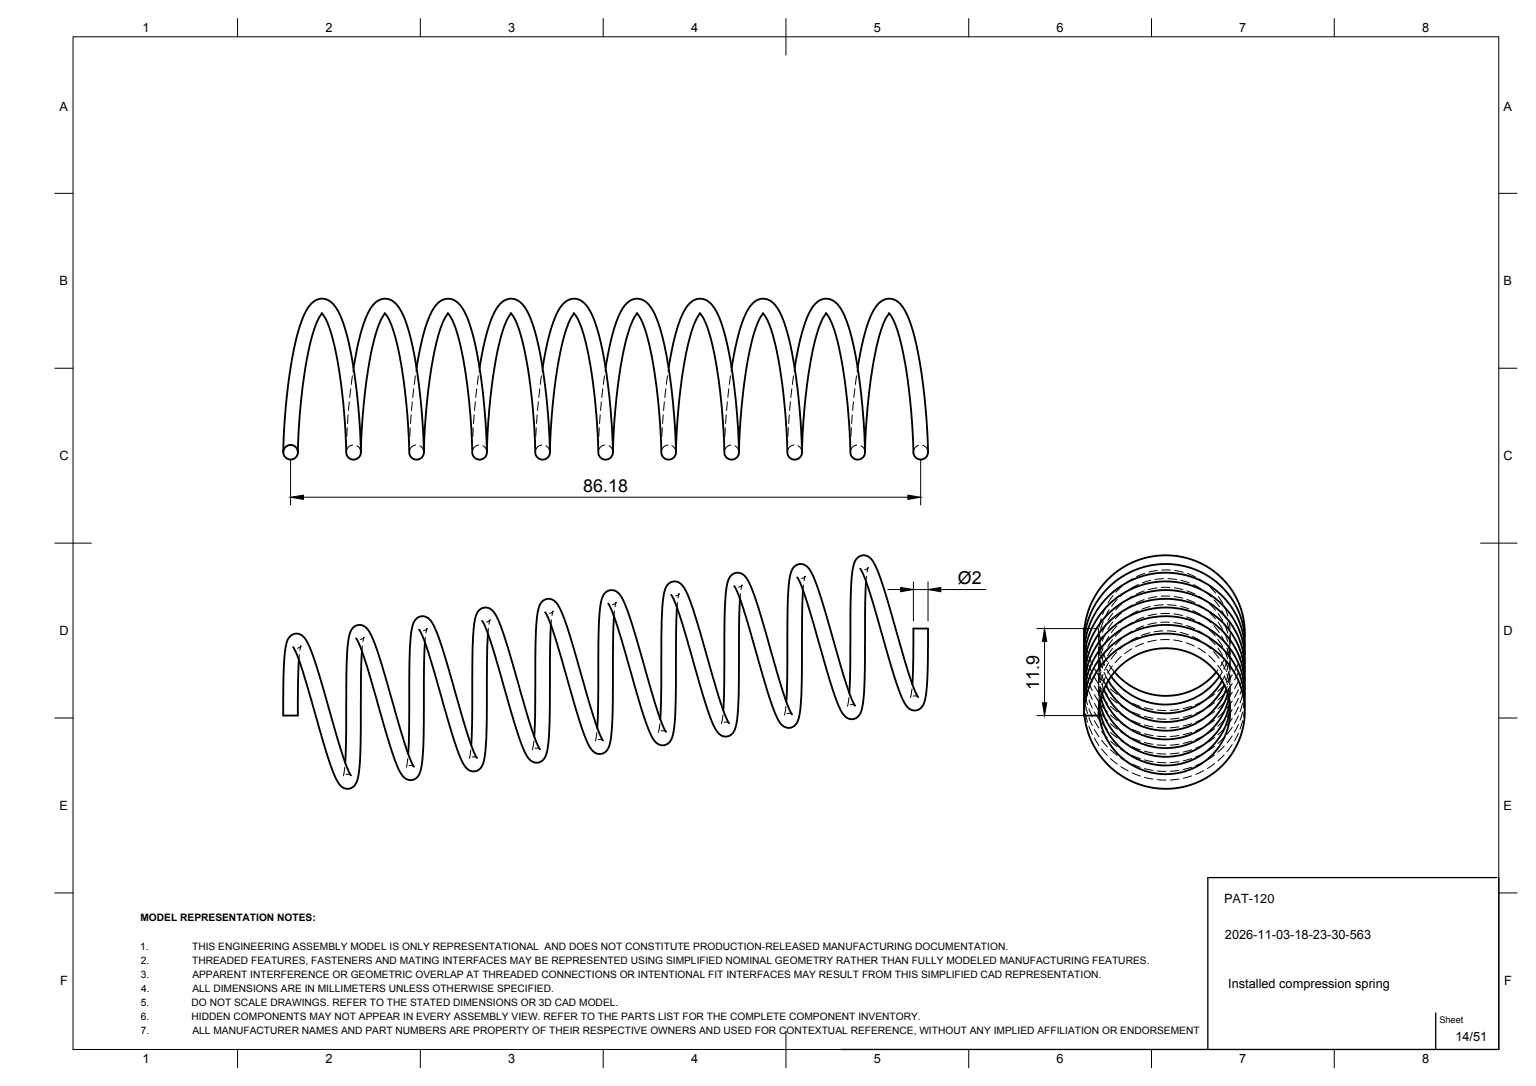
ISO-10303-21;
HEADER;
/* Generated by software containing ST-Developer
 * from STEP Tools, Inc. (www.steptools.com) 
 */

FILE_DESCRIPTION(
/* description */ ('Vibration shaker table dummy'),
/* implementation_level */ '2;1');

FILE_NAME(
/* name */ 'Installed compression spring.step',
/* time_stamp */ '2026-10-27T10:55:14-07:00',
/* author */ (''),
/* organization */ (''),
/* preprocessor_version */ 'ST-DEVELOPER v20.2',
/* originating_system */ 'Autodesk Translation Framework v15.17.0.0',
/* authorisation */ '');

FILE_SCHEMA (('AUTOMOTIVE_DESIGN { 1 0 10303 214 3 1 1 }'));
ENDSEC;

DATA;
#10=MECHANICAL_DESIGN_GEOMETRIC_PRESENTATION_REPRESENTATION('',(#695),#22394);
#586=B_SPLINE_CURVE_WITH_KNOTS('',3,(#15906,#15907,#15908,#15909,#15910,
#15911,#15912,#15913,#15914,#15915,#15916,#15917,#15918,#15919,#15920,#15921,
#15922,#15923,#15924,#15925,#15926,#15927,#15928,#15929,#15930,#15931,#15932,
#15933,#15934,#15935,#15936,#15937,#15938,#15939,#15940,#15941,#15942,#15943,
#15944,#15945,#15946,#15947,#15948,#15949,#15950,#15951,#15952,#15953,#15954,
#15955,#15956,#15957,#15958,#15959,#15960,#15961,#15962,#15963,#15964,#15965,
#15966,#15967,#15968,#15969,#15970,#15971,#15972,#15973,#15974,#15975,#15976,
#15977,#15978,#15979,#15980,#15981,#15982,#15983,#15984,#15985,#15986,#15987,
#15988,#15989,#15990,#15991,#15992,#15993,#15994,#15995,#15996,#15997,#15998,
#15999,#16000,#16001,#16002,#16003,#16004,#16005,#16006,#16007,#16008,#16009,
#16010,#16011,#16012,#16013,#16014,#16015,#16016,#16017,#16018,#16019,#16020,
#16021,#16022,#16023,#16024,#16025,#16026,#16027,#16028,#16029,#16030,#16031,
#16032,#16033,#16034,#16035,#16036,#16037,#16038,#16039),.UNSPECIFIED.,
 .F.,.F.,(4,1,1,1,1,1,1,1,1,1,1,1,1,1,1,1,1,1,1,1,1,1,1,1,1,1,1,1,1,1,1,
1,1,1,1,1,1,1,1,1,1,1,1,1,1,1,1,1,1,1,1,1,1,1,1,1,1,1,1,1,1,1,1,1,1,1,1,
1,1,1,1,1,1,1,1,1,1,1,1,1,1,1,1,1,1,1,1,1,1,1,1,1,1,1,1,1,1,1,1,1,1,1,1,
1,1,1,1,1,1,1,1,1,1,1,1,1,1,1,1,1,1,1,1,1,1,1,1,1,1,1,1,4),(0.,0.00892857142857143,
0.0178571428571429,0.0267857142857143,0.0357142857142857,0.0446428571428571,
0.0535714285714286,0.0625,0.0714285714285714,0.0803571428571428,0.0892857142857143,
0.0982142857142857,0.107142857142857,0.116071428571429,0.125,0.133928571428571,
0.142857142857143,0.150793650793651,0.154761904761905,0.156746031746032,
0.158730158730159,0.166666666666667,0.174603174603175,0.182539682539683,
0.19047619047619,0.196428571428571,0.202380952380952,0.208333333333333,
0.214285714285714,0.222222222222222,0.23015873015873,0.238095238095238,
0.241071428571429,0.244047619047619,0.25,0.255952380952381,0.261904761904762,
0.267857142857143,0.273809523809524,0.279761904761905,0.285714285714286,
0.297619047619048,0.30952380952381,0.321428571428571,0.327380952380952,
0.333333333333333,0.341269841269841,0.349206349206349,0.357142857142857,
0.365079365079365,0.373015873015873,0.380952380952381,0.386904761904762,
0.392857142857143,0.398809523809524,0.404761904761905,0.410714285714286,
0.416666666666667,0.422619047619048,0.428571428571429,0.4375,0.446428571428571,
0.455357142857143,0.459821428571429,0.464285714285714,0.470238095238095,
0.482142857142857,0.491071428571429,0.5,0.508928571428571,0.517857142857143,
0.526785714285714,0.535714285714286,0.544642857142857,0.553571428571429,
0.5625,0.571428571428571,0.580357142857143,0.589285714285714,0.598214285714286,
0.607142857142857,0.616071428571429,0.625,0.633928571428571,0.638392857142857,
0.642857142857143,0.650793650793651,0.658730158730159,0.666666666666667,
0.672619047619048,0.678571428571428,0.684523809523809,0.69047619047619,
0.696428571428571,0.702380952380952,0.708333333333333,0.714285714285714,
0.720238095238095,0.726190476190476,0.732142857142857,0.738095238095238,
0.744047619047619,0.75,0.755952380952381,0.761904761904762,0.76984126984127,
0.777777777777778,0.785714285714286,0.794642857142857,0.803571428571428,
0.8125,0.821428571428571,0.830357142857143,0.839285714285714,0.848214285714286,
0.857142857142857,0.866071428571429,0.875,0.883928571428571,0.892857142857143,
0.901785714285714,0.910714285714286,0.919642857142857,0.928571428571429,
0.9375,0.946428571428571,0.955357142857143,0.964285714285714,0.973214285714286,
0.982142857142857,0.991071428571429,1.),.UNSPECIFIED.);
#590=B_SPLINE_SURFACE_WITH_KNOTS('',3,3,((#14563,#14564,#14565,#14566,#14567,
#14568,#14569,#14570,#14571,#14572,#14573,#14574,#14575,#14576,#14577,#14578,
#14579,#14580,#14581,#14582,#14583,#14584,#14585,#14586,#14587,#14588,#14589,
#14590,#14591,#14592,#14593,#14594,#14595,#14596,#14597,#14598,#14599,#14600,
#14601,#14602,#14603,#14604,#14605,#14606,#14607,#14608,#14609,#14610,#14611,
#14612,#14613,#14614,#14615,#14616,#14617,#14618,#14619,#14620,#14621,#14622,
#14623,#14624,#14625,#14626,#14627,#14628,#14629,#14630,#14631,#14632,#14633,
#14634,#14635,#14636,#14637,#14638,#14639,#14640,#14641,#14642,#14643,#14644,
#14645,#14646,#14647,#14648,#14649,#14650,#14651,#14652,#14653,#14654,#14655,
#14656,#14657,#14658,#14659,#14660,#14661,#14662,#14663,#14664,#14665,#14666,
#14667,#14668,#14669,#14670,#14671,#14672,#14673,#14674,#14675,#14676,#14677,
#14678,#14679,#14680,#14681,#14682,#14683,#14684,#14685,#14686,#14687,#14688,
#14689,#14690,#14691,#14692,#14693,#14694,#14695,#14696),(#14697,#14698,
#14699,#14700,#14701,#14702,#14703,#14704,#14705,#14706,#14707,#14708,#14709,
#14710,#14711,#14712,#14713,#14714,#14715,#14716,#14717,#14718,#14719,#14720,
#14721,#14722,#14723,#14724,#14725,#14726,#14727,#14728,#14729,#14730,#14731,
#14732,#14733,#14734,#14735,#14736,#14737,#14738,#14739,#14740,#14741,#14742,
#14743,#14744,#14745,#14746,#14747,#14748,#14749,#14750,#14751,#14752,#14753,
#14754,#14755,#14756,#14757,#14758,#14759,#14760,#14761,#14762,#14763,#14764,
#14765,#14766,#14767,#14768,#14769,#14770,#14771,#14772,#14773,#14774,#14775,
#14776,#14777,#14778,#14779,#14780,#14781,#14782,#14783,#14784,#14785,#14786,
#14787,#14788,#14789,#14790,#14791,#14792,#14793,#14794,#14795,#14796,#14797,
#14798,#14799,#14800,#14801,#14802,#14803,#14804,#14805,#14806,#14807,#14808,
#14809,#14810,#14811,#14812,#14813,#14814,#14815,#14816,#14817,#14818,#14819,
#14820,#14821,#14822,#14823,#14824,#14825,#14826,#14827,#14828,#14829,#14830),
(#14831,#14832,#14833,#14834,#14835,#14836,#14837,#14838,#14839,#14840,
#14841,#14842,#14843,#14844,#14845,#14846,#14847,#14848,#14849,#14850,#14851,
#14852,#14853,#14854,#14855,#14856,#14857,#14858,#14859,#14860,#14861,#14862,
#14863,#14864,#14865,#14866,#14867,#14868,#14869,#14870,#14871,#14872,#14873,
#14874,#14875,#14876,#14877,#14878,#14879,#14880,#14881,#14882,#14883,#14884,
#14885,#14886,#14887,#14888,#14889,#14890,#14891,#14892,#14893,#14894,#14895,
#14896,#14897,#14898,#14899,#14900,#14901,#14902,#14903,#14904,#14905,#14906,
#14907,#14908,#14909,#14910,#14911,#14912,#14913,#14914,#14915,#14916,#14917,
#14918,#14919,#14920,#14921,#14922,#14923,#14924,#14925,#14926,#14927,#14928,
#14929,#14930,#14931,#14932,#14933,#14934,#14935,#14936,#14937,#14938,#14939,
#14940,#14941,#14942,#14943,#14944,#14945,#14946,#14947,#14948,#14949,#14950,
#14951,#14952,#14953,#14954,#14955,#14956,#14957,#14958,#14959,#14960,#14961,
#14962,#14963,#14964),(#14965,#14966,#14967,#14968,#14969,#14970,#14971,
#14972,#14973,#14974,#14975,#14976,#14977,#14978,#14979,#14980,#14981,#14982,
#14983,#14984,#14985,#14986,#14987,#14988,#14989,#14990,#14991,#14992,#14993,
#14994,#14995,#14996,#14997,#14998,#14999,#15000,#15001,#15002,#15003,#15004,
#15005,#15006,#15007,#15008,#15009,#15010,#15011,#15012,#15013,#15014,#15015,
#15016,#15017,#15018,#15019,#15020,#15021,#15022,#15023,#15024,#15025,#15026,
#15027,#15028,#15029,#15030,#15031,#15032,#15033,#15034,#15035,#15036,#15037,
#15038,#15039,#15040,#15041,#15042,#15043,#15044,#15045,#15046,#15047,#15048,
#15049,#15050,#15051,#15052,#15053,#15054,#15055,#15056,#15057,#15058,#15059,
#15060,#15061,#15062,#15063,#15064,#15065,#15066,#15067,#15068,#15069,#15070,
#15071,#15072,#15073,#15074,#15075,#15076,#15077,#15078,#15079,#15080,#15081,
#15082,#15083,#15084,#15085,#15086,#15087,#15088,#15089,#15090,#15091,#15092,
#15093,#15094,#15095,#15096,#15097,#15098),(#15099,#15100,#15101,#15102,
#15103,#15104,#15105,#15106,#15107,#15108,#15109,#15110,#15111,#15112,#15113,
#15114,#15115,#15116,#15117,#15118,#15119,#15120,#15121,#15122,#15123,#15124,
#15125,#15126,#15127,#15128,#15129,#15130,#15131,#15132,#15133,#15134,#15135,
#15136,#15137,#15138,#15139,#15140,#15141,#15142,#15143,#15144,#15145,#15146,
#15147,#15148,#15149,#15150,#15151,#15152,#15153,#15154,#15155,#15156,#15157,
#15158,#15159,#15160,#15161,#15162,#15163,#15164,#15165,#15166,#15167,#15168,
#15169,#15170,#15171,#15172,#15173,#15174,#15175,#15176,#15177,#15178,#15179,
#15180,#15181,#15182,#15183,#15184,#15185,#15186,#15187,#15188,#15189,#15190,
#15191,#15192,#15193,#15194,#15195,#15196,#15197,#15198,#15199,#15200,#15201,
#15202,#15203,#15204,#15205,#15206,#15207,#15208,#15209,#15210,#15211,#15212,
#15213,#15214,#15215,#15216,#15217,#15218,#15219,#15220,#15221,#15222,#15223,
#15224,#15225,#15226,#15227,#15228,#15229,#15230,#15231,#15232),(#15233,
#15234,#15235,#15236,#15237,#15238,#15239,#15240,#15241,#15242,#15243,#15244,
#15245,#15246,#15247,#15248,#15249,#15250,#15251,#15252,#15253,#15254,#15255,
#15256,#15257,#15258,#15259,#15260,#15261,#15262,#15263,#15264,#15265,#15266,
#15267,#15268,#15269,#15270,#15271,#15272,#15273,#15274,#15275,#15276,#15277,
#15278,#15279,#15280,#15281,#15282,#15283,#15284,#15285,#15286,#15287,#15288,
#15289,#15290,#15291,#15292,#15293,#15294,#15295,#15296,#15297,#15298,#15299,
#15300,#15301,#15302,#15303,#15304,#15305,#15306,#15307,#15308,#15309,#15310,
#15311,#15312,#15313,#15314,#15315,#15316,#15317,#15318,#15319,#15320,#15321,
#15322,#15323,#15324,#15325,#15326,#15327,#15328,#15329,#15330,#15331,#15332,
#15333,#15334,#15335,#15336,#15337,#15338,#15339,#15340,#15341,#15342,#15343,
#15344,#15345,#15346,#15347,#15348,#15349,#15350,#15351,#15352,#15353,#15354,
#15355,#15356,#15357,#15358,#15359,#15360,#15361,#15362,#15363,#15364,#15365,
#15366),(#15367,#15368,#15369,#15370,#15371,#15372,#15373,#15374,#15375,
#15376,#15377,#15378,#15379,#15380,#15381,#15382,#15383,#15384,#15385,#15386,
#15387,#15388,#15389,#15390,#15391,#15392,#15393,#15394,#15395,#15396,#15397,
#15398,#15399,#15400,#15401,#15402,#15403,#15404,#15405,#15406,#15407,#15408,
#15409,#15410,#15411,#15412,#15413,#15414,#15415,#15416,#15417,#15418,#15419,
#15420,#15421,#15422,#15423,#15424,#15425,#15426,#15427,#15428,#15429,#15430,
#15431,#15432,#15433,#15434,#15435,#15436,#15437,#15438,#15439,#15440,#15441,
#15442,#15443,#15444,#15445,#15446,#15447,#15448,#15449,#15450,#15451,#15452,
#15453,#15454,#15455,#15456,#15457,#15458,#15459,#15460,#15461,#15462,#15463,
#15464,#15465,#15466,#15467,#15468,#15469,#15470,#15471,#15472,#15473,#15474,
#15475,#15476,#15477,#15478,#15479,#15480,#15481,#15482,#15483,#15484,#15485,
#15486,#15487,#15488,#15489,#15490,#15491,#15492,#15493,#15494,#15495,#15496,
#15497,#15498,#15499,#15500),(#15501,#15502,#15503,#15504,#15505,#15506,
#15507,#15508,#15509,#15510,#15511,#15512,#15513,#15514,#15515,#15516,#15517,
#15518,#15519,#15520,#15521,#15522,#15523,#15524,#15525,#15526,#15527,#15528,
#15529,#15530,#15531,#15532,#15533,#15534,#15535,#15536,#15537,#15538,#15539,
#15540,#15541,#15542,#15543,#15544,#15545,#15546,#15547,#15548,#15549,#15550,
#15551,#15552,#15553,#15554,#15555,#15556,#15557,#15558,#15559,#15560,#15561,
#15562,#15563,#15564,#15565,#15566,#15567,#15568,#15569,#15570,#15571,#15572,
#15573,#15574,#15575,#15576,#15577,#15578,#15579,#15580,#15581,#15582,#15583,
#15584,#15585,#15586,#15587,#15588,#15589,#15590,#15591,#15592,#15593,#15594,
#15595,#15596,#15597,#15598,#15599,#15600,#15601,#15602,#15603,#15604,#15605,
#15606,#15607,#15608,#15609,#15610,#15611,#15612,#15613,#15614,#15615,#15616,
#15617,#15618,#15619,#15620,#15621,#15622,#15623,#15624,#15625,#15626,#15627,
#15628,#15629,#15630,#15631,#15632,#15633,#15634),(#15635,#15636,#15637,
#15638,#15639,#15640,#15641,#15642,#15643,#15644,#15645,#15646,#15647,#15648,
#15649,#15650,#15651,#15652,#15653,#15654,#15655,#15656,#15657,#15658,#15659,
#15660,#15661,#15662,#15663,#15664,#15665,#15666,#15667,#15668,#15669,#15670,
#15671,#15672,#15673,#15674,#15675,#15676,#15677,#15678,#15679,#15680,#15681,
#15682,#15683,#15684,#15685,#15686,#15687,#15688,#15689,#15690,#15691,#15692,
#15693,#15694,#15695,#15696,#15697,#15698,#15699,#15700,#15701,#15702,#15703,
#15704,#15705,#15706,#15707,#15708,#15709,#15710,#15711,#15712,#15713,#15714,
#15715,#15716,#15717,#15718,#15719,#15720,#15721,#15722,#15723,#15724,#15725,
#15726,#15727,#15728,#15729,#15730,#15731,#15732,#15733,#15734,#15735,#15736,
#15737,#15738,#15739,#15740,#15741,#15742,#15743,#15744,#15745,#15746,#15747,
#15748,#15749,#15750,#15751,#15752,#15753,#15754,#15755,#15756,#15757,#15758,
#15759,#15760,#15761,#15762,#15763,#15764,#15765,#15766,#15767,#15768),
(#15769,#15770,#15771,#15772,#15773,#15774,#15775,#15776,#15777,#15778,
#15779,#15780,#15781,#15782,#15783,#15784,#15785,#15786,#15787,#15788,#15789,
#15790,#15791,#15792,#15793,#15794,#15795,#15796,#15797,#15798,#15799,#15800,
#15801,#15802,#15803,#15804,#15805,#15806,#15807,#15808,#15809,#15810,#15811,
#15812,#15813,#15814,#15815,#15816,#15817,#15818,#15819,#15820,#15821,#15822,
#15823,#15824,#15825,#15826,#15827,#15828,#15829,#15830,#15831,#15832,#15833,
#15834,#15835,#15836,#15837,#15838,#15839,#15840,#15841,#15842,#15843,#15844,
#15845,#15846,#15847,#15848,#15849,#15850,#15851,#15852,#15853,#15854,#15855,
#15856,#15857,#15858,#15859,#15860,#15861,#15862,#15863,#15864,#15865,#15866,
#15867,#15868,#15869,#15870,#15871,#15872,#15873,#15874,#15875,#15876,#15877,
#15878,#15879,#15880,#15881,#15882,#15883,#15884,#15885,#15886,#15887,#15888,
#15889,#15890,#15891,#15892,#15893,#15894,#15895,#15896,#15897,#15898,#15899,
#15900,#15901,#15902)),.UNSPECIFIED.,.T.,.F.,.F.,(4,1,1,1,1,1,1,4),(4,1,
1,1,1,1,1,1,1,1,1,1,1,1,1,1,1,1,1,1,1,1,1,1,1,1,1,1,1,1,1,1,1,1,1,1,1,1,
1,1,1,1,1,1,1,1,1,1,1,1,1,1,1,1,1,1,1,1,1,1,1,1,1,1,1,1,1,1,1,1,1,1,1,1,
1,1,1,1,1,1,1,1,1,1,1,1,1,1,1,1,1,1,1,1,1,1,1,1,1,1,1,1,1,1,1,1,1,1,1,1,
1,1,1,1,1,1,1,1,1,1,1,1,1,1,1,1,1,1,1,1,1,4),(-3.14159265358979,-2.24399475256414,
-1.34639685153848,-0.448798950512828,0.448798950512828,1.34639685153848,
2.24399475256414,3.14159265358979),(0.,0.00892857142857143,0.0178571428571429,
0.0267857142857143,0.0357142857142857,0.0446428571428571,0.0535714285714286,
0.0625,0.0714285714285714,0.0803571428571428,0.0892857142857143,0.0982142857142857,
0.107142857142857,0.116071428571429,0.125,0.133928571428571,0.142857142857143,
0.150793650793651,0.154761904761905,0.156746031746032,0.158730158730159,
0.166666666666667,0.174603174603175,0.182539682539683,0.19047619047619,
0.196428571428571,0.202380952380952,0.208333333333333,0.214285714285714,
0.222222222222222,0.23015873015873,0.238095238095238,0.241071428571429,
0.244047619047619,0.25,0.255952380952381,0.261904761904762,0.267857142857143,
0.273809523809524,0.279761904761905,0.285714285714286,0.297619047619048,
0.30952380952381,0.321428571428571,0.327380952380952,0.333333333333333,
0.341269841269841,0.349206349206349,0.357142857142857,0.365079365079365,
0.373015873015873,0.380952380952381,0.386904761904762,0.392857142857143,
0.398809523809524,0.404761904761905,0.410714285714286,0.416666666666667,
0.422619047619048,0.428571428571429,0.4375,0.446428571428571,0.455357142857143,
0.459821428571429,0.464285714285714,0.470238095238095,0.482142857142857,
0.491071428571429,0.5,0.508928571428571,0.517857142857143,0.526785714285714,
0.535714285714286,0.544642857142857,0.553571428571429,0.5625,0.571428571428571,
0.580357142857143,0.589285714285714,0.598214285714286,0.607142857142857,
0.616071428571429,0.625,0.633928571428571,0.638392857142857,0.642857142857143,
0.650793650793651,0.658730158730159,0.666666666666667,0.672619047619048,
0.678571428571428,0.684523809523809,0.69047619047619,0.696428571428571,
0.702380952380952,0.708333333333333,0.714285714285714,0.720238095238095,
0.726190476190476,0.732142857142857,0.738095238095238,0.744047619047619,
0.75,0.755952380952381,0.761904761904762,0.76984126984127,0.777777777777778,
0.785714285714286,0.794642857142857,0.803571428571428,0.8125,0.821428571428571,
0.830357142857143,0.839285714285714,0.848214285714286,0.857142857142857,
0.866071428571429,0.875,0.883928571428571,0.892857142857143,0.901785714285714,
0.910714285714286,0.919642857142857,0.928571428571429,0.9375,0.946428571428571,
0.955357142857143,0.964285714285714,0.973214285714286,0.982142857142857,
0.991071428571429,1.),.UNSPECIFIED.);
#603=SHAPE_REPRESENTATION_RELATIONSHIP('SRR','None',#22649,#649);
#649=ADVANCED_BREP_SHAPE_REPRESENTATION('',(#741),#22355);
#695=STYLED_ITEM('',(#22961),#741);
#741=MANIFOLD_SOLID_BREP('Body1',#9213);
#1124=PLANE('',#10016);
#1125=PLANE('',#10017);
#1463=FACE_OUTER_BOUND('',#2063,.T.);
#1464=FACE_OUTER_BOUND('',#2064,.T.);
#1465=FACE_OUTER_BOUND('',#2065,.T.);
#2063=EDGE_LOOP('',(#6822,#6823,#6824,#6825));
#2064=EDGE_LOOP('',(#6826));
#2065=EDGE_LOOP('',(#6827));
#3980=CIRCLE('',#10014,0.1);
#3981=CIRCLE('',#10015,0.1);
#4559=VERTEX_POINT('',#15903);
#4560=VERTEX_POINT('',#15905);
#5404=EDGE_CURVE('',#4559,#4559,#3980,.T.);
#5405=EDGE_CURVE('',#4559,#4560,#586,.T.);
#5406=EDGE_CURVE('',#4560,#4560,#3981,.T.);
#6822=ORIENTED_EDGE('',*,*,#5404,.T.);
#6823=ORIENTED_EDGE('',*,*,#5405,.T.);
#6824=ORIENTED_EDGE('',*,*,#5406,.F.);
#6825=ORIENTED_EDGE('',*,*,#5405,.F.);
#6826=ORIENTED_EDGE('',*,*,#5406,.T.);
#6827=ORIENTED_EDGE('',*,*,#5404,.F.);
#8828=ADVANCED_FACE('',(#1463),#590,.T.);
#8829=ADVANCED_FACE('',(#1464),#1124,.T.);
#8830=ADVANCED_FACE('',(#1465),#1125,.F.);
#9213=CLOSED_SHELL('',(#8828,#8829,#8830));
#10013=AXIS2_PLACEMENT_3D('',#14562,#11624,#11625);
#10014=AXIS2_PLACEMENT_3D('',#15904,#11626,#11627);
#10015=AXIS2_PLACEMENT_3D('',#16040,#11628,#11629);
#10016=AXIS2_PLACEMENT_3D('',#16041,#11630,#11631);
#10017=AXIS2_PLACEMENT_3D('',#16042,#11632,#11633);
#11624=DIRECTION('axis',(0.,0.,1.));
#11625=DIRECTION('refdir',(1.,0.,0.));
#11626=DIRECTION('center_axis',(-0.000133356290274077,0.990604928518996,
0.136754735969086));
#11627=DIRECTION('ref_axis',(1.84100680060121E-5,-0.136754734729895,0.990604937495279));
#11628=DIRECTION('center_axis',(0.000133356194773129,0.99060492849245,0.136754736161472));
#11629=DIRECTION('ref_axis',(-0.722226697925938,0.0946826990450871,-0.685145081938514));
#11630=DIRECTION('center_axis',(0.000133356194773129,0.99060492849245,0.136754736161472));
#11631=DIRECTION('ref_axis',(-0.722226697925938,0.0946826990450871,-0.685145081938514));
#11632=DIRECTION('center_axis',(-0.000133356290274077,0.990604928518996,
0.136754735969086));
#11633=DIRECTION('ref_axis',(1.84100680060121E-5,-0.136754734729895,0.990604937495279));
#14562=CARTESIAN_POINT('',(0.,0.,0.));
#14563=CARTESIAN_POINT('Ctrl Pts',(-5.0000018410068,-3.98632452652701,2.60093950625047));
#14564=CARTESIAN_POINT('Ctrl Pts',(-5.00002711936198,-3.79855038268961,
2.62686205390092));
#14565=CARTESIAN_POINT('Ctrl Pts',(-5.10766548646186,-3.42414266353048,
2.67881373981085));
#14566=CARTESIAN_POINT('Ctrl Pts',(-5.54728618664091,-3.02997941177219,
2.75738438838345));
#14567=CARTESIAN_POINT('Ctrl Pts',(-6.13328094577175,-2.93005881251319,
2.83651316903494));
#14568=CARTESIAN_POINT('Ctrl Pts',(-6.68670283260197,-3.15858336118752,
2.91622304878198));
#14569=CARTESIAN_POINT('Ctrl Pts',(-7.03616187921695,-3.65012597802659,
2.99648821676135));
#14570=CARTESIAN_POINT('Ctrl Pts',(-7.07062949516082,-4.25616589762635,
3.07729930317819));
#14571=CARTESIAN_POINT('Ctrl Pts',(-6.77580863517498,-4.79139923899731,
3.15863489698049));
#14572=CARTESIAN_POINT('Ctrl Pts',(-6.23777999713871,-5.08919902934938,
3.24047455745509));
#14573=CARTESIAN_POINT('Ctrl Pts',(-5.62032344264714,-5.05504677509261,
3.32279321070673));
#14574=CARTESIAN_POINT('Ctrl Pts',(-5.11287137916696,-4.69557478020053,
3.40556356877954));
#14575=CARTESIAN_POINT('Ctrl Pts',(-4.87329914702911,-4.11831903637453,
3.48875540125931));
#14576=CARTESIAN_POINT('Ctrl Pts',(-4.97807346419814,-3.49920456570944,
3.57233609900605));
#14577=CARTESIAN_POINT('Ctrl Pts',(-5.39799493781825,-3.02877333945258,
3.65627071903615));
#14578=CARTESIAN_POINT('Ctrl Pts',(-6.00610273172108,-2.85326324045065,
3.74052224127624));
#14579=CARTESIAN_POINT('Ctrl Pts',(-6.61643757836359,-3.02876545098225,
3.82505176791358));
#14580=CARTESIAN_POINT('Ctrl Pts',(-7.02513160270699,-3.48597574268572,
3.90667922493066));
#14581=CARTESIAN_POINT('Ctrl Pts',(-7.12235641775929,-3.9685483460108,3.97275270898905));
#14582=CARTESIAN_POINT('Ctrl Pts',(-7.06636481269846,-4.28466100128236,
4.01685604551847));
#14583=CARTESIAN_POINT('Ctrl Pts',(-7.00182040328561,-4.45530975229043,
4.04207155819959));
#14584=CARTESIAN_POINT('Ctrl Pts',(-6.87402691871924,-4.69744869614318,
4.07990746733096));
#14585=CARTESIAN_POINT('Ctrl Pts',(-6.57124878899927,-4.99309357202046,
4.1367051149187));
#14586=CARTESIAN_POINT('Ctrl Pts',(-6.02768033690931,-5.14605913758532,
4.2124974864954));
#14587=CARTESIAN_POINT('Ctrl Pts',(-5.47679456345111,-5.0204436702095,4.28832048286543));
#14588=CARTESIAN_POINT('Ctrl Pts',(-5.08889541312948,-4.67743201497751,
4.35782392862843));
#14589=CARTESIAN_POINT('Ctrl Pts',(-4.90355272665998,-4.25185719379132,
4.42098501738742));
#14590=CARTESIAN_POINT('Ctrl Pts',(-4.88772422317122,-3.83457870292561,
4.47779828347438));
#14591=CARTESIAN_POINT('Ctrl Pts',(-5.02577825319216,-3.44096047951616,
4.5345666000236));
#14592=CARTESIAN_POINT('Ctrl Pts',(-5.32758243531257,-3.08955719770179,
4.59757801626674));
#14593=CARTESIAN_POINT('Ctrl Pts',(-5.79757132369034,-2.87764760865861,
4.66678930745632));
#14594=CARTESIAN_POINT('Ctrl Pts',(-6.35748141231083,-2.91980778121556,
4.74213608943437));
#14595=CARTESIAN_POINT('Ctrl Pts',(-6.72958410590507,-3.16055362161142,
4.80163845366161));
#14596=CARTESIAN_POINT('Ctrl Pts',(-6.922583408066,-3.41255717151317,4.8453962925926));
#14597=CARTESIAN_POINT('Ctrl Pts',(-7.04520229026909,-3.65506744231538,
4.88286085267916));
#14598=CARTESIAN_POINT('Ctrl Pts',(-7.10903827020174,-3.9926759490213,4.92960885619655));
#14599=CARTESIAN_POINT('Ctrl Pts',(-7.032354492376,-4.39667067923105,4.98556279568034));
#14600=CARTESIAN_POINT('Ctrl Pts',(-6.81415974257675,-4.74396102273289,
5.04136211338037));
#14601=CARTESIAN_POINT('Ctrl Pts',(-6.48510242262688,-4.98648342248571,
5.09699623581333));
#14602=CARTESIAN_POINT('Ctrl Pts',(-6.09122164110091,-5.09213718968761,
5.15245506498449));
#14603=CARTESIAN_POINT('Ctrl Pts',(-5.6879156360413,-5.04618557814476,5.20772889788153));
#14604=CARTESIAN_POINT('Ctrl Pts',(-5.20960410281967,-4.79482820495352,
5.28116853491036));
#14605=CARTESIAN_POINT('Ctrl Pts',(-4.85635661256684,-4.18339627204868,
5.37246079310469));
#14606=CARTESIAN_POINT('Ctrl Pts',(-5.04534497366866,-3.36152922837358,
5.4811368047244));
#14607=CARTESIAN_POINT('Ctrl Pts',(-5.62045222073828,-2.97210695679973,
5.57092649482181));
#14608=CARTESIAN_POINT('Ctrl Pts',(-6.14491401311764,-2.95446524901901,
5.64227218329944));
#14609=CARTESIAN_POINT('Ctrl Pts',(-6.55538629310792,-3.09741218079302,
5.70145206897501));
#14610=CARTESIAN_POINT('Ctrl Pts',(-6.90061904209687,-3.43455608810828,
5.76619150175189));
#14611=CARTESIAN_POINT('Ctrl Pts',(-7.05403180026006,-3.93434682913999,
5.83636208061574));
#14612=CARTESIAN_POINT('Ctrl Pts',(-6.95084370870626,-4.44331194962687,
5.90607316768221));
#14613=CARTESIAN_POINT('Ctrl Pts',(-6.61884201115902,-4.83828819326241,
5.97532164622816));
#14614=CARTESIAN_POINT('Ctrl Pts',(-6.14163977231472,-5.02507153362565,
6.04410658214742));
#14615=CARTESIAN_POINT('Ctrl Pts',(-5.67874308979945,-4.96670943531882,
6.10673565115305));
#14616=CARTESIAN_POINT('Ctrl Pts',(-5.32673727495899,-4.74487796933182,
6.16333654805419));
#14617=CARTESIAN_POINT('Ctrl Pts',(-5.10557737295403,-4.44521639081723,
6.21402149420468));
#14618=CARTESIAN_POINT('Ctrl Pts',(-5.00986236436416,-4.08706033297606,
6.26445344628883));
#14619=CARTESIAN_POINT('Ctrl Pts',(-5.05132140869747,-3.72058500062059,
6.31463598386295));
#14620=CARTESIAN_POINT('Ctrl Pts',(-5.22295427342147,-3.39619318419661,
6.36457331207659));
#14621=CARTESIAN_POINT('Ctrl Pts',(-5.49996349858563,-3.15797332202467,
6.41427030413784));
#14622=CARTESIAN_POINT('Ctrl Pts',(-5.843023257891,-3.03825996963253,6.46373244033231));
#14623=CARTESIAN_POINT('Ctrl Pts',(-6.2651798733637,-3.05368284090179,6.52117143934356));
#14624=CARTESIAN_POINT('Ctrl Pts',(-6.69395218073661,-3.29085487418832,
6.58644589644131));
#14625=CARTESIAN_POINT('Ctrl Pts',(-6.9588514090406,-3.77142724594311,6.65940509135759));
#14626=CARTESIAN_POINT('Ctrl Pts',(-6.93289301903251,-4.22410112506723,
6.71983222544231));
#14627=CARTESIAN_POINT('Ctrl Pts',(-6.77106481048377,-4.53615877260298,
6.76796591761938));
#14628=CARTESIAN_POINT('Ctrl Pts',(-6.57088599598262,-4.74749645053629,
6.8079662999785));
#14629=CARTESIAN_POINT('Ctrl Pts',(-6.18196007039062,-4.95496402481898,
6.86778079666891));
#14630=CARTESIAN_POINT('Ctrl Pts',(-5.63200940413013,-4.91297894303413,
6.93919834468442));
#14631=CARTESIAN_POINT('Ctrl Pts',(-5.18963313111942,-4.51545599119052,
7.01814869825501));
#14632=CARTESIAN_POINT('Ctrl Pts',(-5.04266994609727,-4.00519996765647,
7.08893288548598));
#14633=CARTESIAN_POINT('Ctrl Pts',(-5.18994160065279,-3.49569082009585,
7.15948665627275));
#14634=CARTESIAN_POINT('Ctrl Pts',(-5.58406477811046,-3.14370617953113,
7.22985222522876));
#14635=CARTESIAN_POINT('Ctrl Pts',(-6.10419876841606,-3.05543002721108,
7.30007283323036));
#14636=CARTESIAN_POINT('Ctrl Pts',(-6.59085610258569,-3.25712241290123,
7.37019262147636));
#14637=CARTESIAN_POINT('Ctrl Pts',(-6.8952969281062,-3.68642062054244,7.44025632508636));
#14638=CARTESIAN_POINT('Ctrl Pts',(-6.92507910037993,-4.2118623997588,7.51030900497373));
#14639=CARTESIAN_POINT('Ctrl Pts',(-6.67029196164112,-4.6727438878236,7.58039577683535));
#14640=CARTESIAN_POINT('Ctrl Pts',(-6.20902606294958,-4.92782413963266,
7.65056157433059));
#14641=CARTESIAN_POINT('Ctrl Pts',(-5.68175068955988,-4.89838259463549,
7.72085085746158));
#14642=CARTESIAN_POINT('Ctrl Pts',(-5.24995696526907,-4.59224234497362,
7.79130734612191));
#14643=CARTESIAN_POINT('Ctrl Pts',(-5.04653976812282,-4.10189023096155,
7.86197377554524));
#14644=CARTESIAN_POINT('Ctrl Pts',(-5.13553771446182,-3.57654536818086,
7.93289164421975));
#14645=CARTESIAN_POINT('Ctrl Pts',(-5.49167958880606,-3.17757206270347,
8.00410097016463));
#14646=CARTESIAN_POINT('Ctrl Pts',(-6.00820878856796,-3.02820291673281,
8.07564000225066));
#14647=CARTESIAN_POINT('Ctrl Pts',(-6.44062187419601,-3.15261370888403,
8.13556092469148));
#14648=CARTESIAN_POINT('Ctrl Pts',(-6.70861130655355,-3.37965195671477,
8.18369776363854));
#14649=CARTESIAN_POINT('Ctrl Pts',(-6.8937105085998,-3.65581236490976,8.22929135600403));
#14650=CARTESIAN_POINT('Ctrl Pts',(-6.97571459288556,-4.05892831151958,
8.28449961702882));
#14651=CARTESIAN_POINT('Ctrl Pts',(-6.83301647708075,-4.52172879570838,
8.34949564023339));
#14652=CARTESIAN_POINT('Ctrl Pts',(-6.51381452164907,-4.83374162454526,
8.40942447333573));
#14653=CARTESIAN_POINT('Ctrl Pts',(-6.13367096105595,-4.96658596055631,
8.46419547642941));
#14654=CARTESIAN_POINT('Ctrl Pts',(-5.77000769054747,-4.95325944490059,
8.51371979160536));
#14655=CARTESIAN_POINT('Ctrl Pts',(-5.43473421944715,-4.80705755452014,
8.56348049202891));
#14656=CARTESIAN_POINT('Ctrl Pts',(-5.17476962038704,-4.5473411130966,8.6134828902317));
#14657=CARTESIAN_POINT('Ctrl Pts',(-5.02691233865341,-4.20890181210803,
8.66373168353468));
#14658=CARTESIAN_POINT('Ctrl Pts',(-5.01287597198371,-3.83802632501149,
8.71423091550292));
#14659=CARTESIAN_POINT('Ctrl Pts',(-5.13588065841094,-3.48587318149708,
8.76498396862734));
#14660=CARTESIAN_POINT('Ctrl Pts',(-5.38027484984219,-3.20156985271231,
8.81599355960519));
#14661=CARTESIAN_POINT('Ctrl Pts',(-5.71337748308179,-3.0254571982762,8.86726173709343));
#14662=CARTESIAN_POINT('Ctrl Pts',(-6.08966550245643,-2.98274869856715,
8.91878984711541));
#14663=CARTESIAN_POINT('Ctrl Pts',(-6.45733798876018,-3.0812109148485,8.97057858675351));
#14664=CARTESIAN_POINT('Ctrl Pts',(-6.76529910592523,-3.30812336168265,
9.02262792849601));
#14665=CARTESIAN_POINT('Ctrl Pts',(-6.96998046112789,-3.63355675694242,
9.07493719450744));
#14666=CARTESIAN_POINT('Ctrl Pts',(-7.04194989283072,-4.01319995364602,
9.12750500078302));
#14667=CARTESIAN_POINT('Ctrl Pts',(-6.96991048459342,-4.39460760383808,
9.18032929219698));
#14668=CARTESIAN_POINT('Ctrl Pts',(-6.73960211403654,-4.76194359718324,
9.23930488555841));
#14669=CARTESIAN_POINT('Ctrl Pts',(-6.33176853957225,-5.02597941464994,
9.30453505646424));
#14670=CARTESIAN_POINT('Ctrl Pts',(-5.79980377218573,-5.06633098935627,
9.37613051632468));
#14671=CARTESIAN_POINT('Ctrl Pts',(-5.29005475531646,-4.836901018808,9.45115010972279));
#14672=CARTESIAN_POINT('Ctrl Pts',(-4.94827191401131,-4.35650564743655,
9.52964181326016));
#14673=CARTESIAN_POINT('Ctrl Pts',(-4.91327405487842,-3.74129847888372,
9.61164803952703));
#14674=CARTESIAN_POINT('Ctrl Pts',(-5.21254904956895,-3.19880095424663,
9.69412425066449));
#14675=CARTESIAN_POINT('Ctrl Pts',(-5.75755518053287,-2.89705290752891,
9.77704206923956));
#14676=CARTESIAN_POINT('Ctrl Pts',(-6.38261532053777,-2.93174547355756,
9.86037047436186));
#14677=CARTESIAN_POINT('Ctrl Pts',(-6.89571246871018,-3.29533246954376,
9.9440760489684));
#14678=CARTESIAN_POINT('Ctrl Pts',(-7.13766462222267,-3.87856431327716,
10.0281231253342));
#14679=CARTESIAN_POINT('Ctrl Pts',(-7.03181307520858,-4.50336859593469,
10.112474009291));
#14680=CARTESIAN_POINT('Ctrl Pts',(-6.60841405754483,-4.9775421382096,10.1970892234063));
#14681=CARTESIAN_POINT('Ctrl Pts',(-5.99601356400164,-5.15419586953956,
10.2819277209876));
#14682=CARTESIAN_POINT('Ctrl Pts',(-5.38220054085499,-4.97753568370925,
10.3669471364924));
#14683=CARTESIAN_POINT('Ctrl Pts',(-4.95580917322647,-4.50058383383181,
10.4521040148979));
#14684=CARTESIAN_POINT('Ctrl Pts',(-4.84845524689304,-3.86918295104257,
10.5373541217208));
#14685=CARTESIAN_POINT('Ctrl Pts',(-5.09367725879538,-3.27712852401529,
10.6226526455382));
#14686=CARTESIAN_POINT('Ctrl Pts',(-5.6163401918585,-2.90630478068196,10.7079544990261));
#14687=CARTESIAN_POINT('Ctrl Pts',(-6.25592072702474,-2.87046899980689,
10.7932145516894));
#14688=CARTESIAN_POINT('Ctrl Pts',(-6.81586294759382,-3.18009679237689,
10.8783879977619));
#14689=CARTESIAN_POINT('Ctrl Pts',(-7.124955642463,-3.73939634942269,10.963430385322));
#14690=CARTESIAN_POINT('Ctrl Pts',(-7.08867264951758,-4.37593520057008,
11.0482983435205));
#14691=CARTESIAN_POINT('Ctrl Pts',(-6.72062823969146,-4.89450906450982,
11.1329488746335));
#14692=CARTESIAN_POINT('Ctrl Pts',(-6.13472454520284,-5.136799701332,11.217341733611));
#14693=CARTESIAN_POINT('Ctrl Pts',(-5.51200536776972,-5.03087324497862,
11.3014349939178));
#14694=CARTESIAN_POINT('Ctrl Pts',(-5.04306930328679,-4.6109089567958,11.3851957518917));
#14695=CARTESIAN_POINT('Ctrl Pts',(-4.92780437314592,-4.2103503377694,11.4407823887583));
#14696=CARTESIAN_POINT('Ctrl Pts',(-4.92777733020741,-4.00946826990451,
11.4685145081939));
#14697=CARTESIAN_POINT('Ctrl Pts',(-5.02992177076987,-3.98632855437981,
2.60093950625047));
#14698=CARTESIAN_POINT('Ctrl Pts',(-5.02994631566211,-3.80400276249367,
2.62610989942328));
#14699=CARTESIAN_POINT('Ctrl Pts',(-5.13440258778751,-3.44058117095201,
2.67653041943034));
#14700=CARTESIAN_POINT('Ctrl Pts',(-5.56132162600835,-3.05771102958624,
2.75283690301094));
#14701=CARTESIAN_POINT('Ctrl Pts',(-6.13074764302092,-2.96056640229043,
2.82972278836909));
#14702=CARTESIAN_POINT('Ctrl Pts',(-6.66896086911222,-3.1827303900304,2.90723424531236));
#14703=CARTESIAN_POINT('Ctrl Pts',(-7.0091712958513,-3.66112442258111,2.98535323605726));
#14704=CARTESIAN_POINT('Ctrl Pts',(-7.04284600518481,-4.25162088811131,
3.06408757941918));
#14705=CARTESIAN_POINT('Ctrl Pts',(-6.75534616813047,-4.77378941641128,
3.14342203482332));
#14706=CARTESIAN_POINT('Ctrl Pts',(-6.22989350052469,-5.06476181444098,
3.22334341795718));
#14707=CARTESIAN_POINT('Ctrl Pts',(-5.62593684855353,-5.03148535851095,
3.3038501203708));
#14708=CARTESIAN_POINT('Ctrl Pts',(-5.1287541466607,-4.67945429549254,3.38491948457682));
#14709=CARTESIAN_POINT('Ctrl Pts',(-4.89355205236567,-4.11311271692517,
3.46653357829839));
#14710=CARTESIAN_POINT('Ctrl Pts',(-4.99637627302549,-3.50458413255717,
3.54866779717306));
#14711=CARTESIAN_POINT('Ctrl Pts',(-5.40970923759118,-3.04128461772533,
3.63129587938778));
#14712=CARTESIAN_POINT('Ctrl Pts',(-6.00950948085903,-2.867992196767,3.71438836781264));
#14713=CARTESIAN_POINT('Ctrl Pts',(-6.61274600784354,-3.04126505973915,
3.79791226147148));
#14714=CARTESIAN_POINT('Ctrl Pts',(-7.01756958403438,-3.49388616164201,
3.87872583853233));
#14715=CARTESIAN_POINT('Ctrl Pts',(-7.1141315386001,-3.97261134085471,3.9442614338042));
#14716=CARTESIAN_POINT('Ctrl Pts',(-7.05852445971495,-4.28666070323465,
3.98807156329228));
#14717=CARTESIAN_POINT('Ctrl Pts',(-6.99436014221873,-4.45631244072124,
4.01313835147944));
#14718=CARTESIAN_POINT('Ctrl Pts',(-6.86726327177174,-4.69714488722618,
4.05076789045709));
#14719=CARTESIAN_POINT('Ctrl Pts',(-6.56590374625076,-4.99156063284653,
4.10729650412945));
#14720=CARTESIAN_POINT('Ctrl Pts',(-6.02371646768625,-5.14428159346822,
4.18289678502633));
#14721=CARTESIAN_POINT('Ctrl Pts',(-5.47318100169159,-5.01887821754281,
4.25865808314083));
#14722=CARTESIAN_POINT('Ctrl Pts',(-5.08477033821112,-4.67558092229865,
4.32822376669194));
#14723=CARTESIAN_POINT('Ctrl Pts',(-4.89886657854121,-4.24885080118007,
4.39155414030818));
#14724=CARTESIAN_POINT('Ctrl Pts',(-4.88291604792826,-3.82987351104406,
4.44859069874469));
#14725=CARTESIAN_POINT('Ctrl Pts',(-5.02168464637103,-3.43409260120211,
4.50566175306661));
#14726=CARTESIAN_POINT('Ctrl Pts',(-5.32548609673626,-3.08026957325351,
4.56909245555632));
#14727=CARTESIAN_POINT('Ctrl Pts',(-5.79936418578429,-2.86648825136964,
4.63887581219755));
#14728=CARTESIAN_POINT('Ctrl Pts',(-6.36494798765252,-2.90895436286898,
4.71498066206858));
#14729=CARTESIAN_POINT('Ctrl Pts',(-6.74144616414175,-3.15244848100526,
4.77515909292762));
#14730=CARTESIAN_POINT('Ctrl Pts',(-6.93695568199013,-3.40771771847224,
4.81948145060093));
#14731=CARTESIAN_POINT('Ctrl Pts',(-7.0612422585727,-3.65351693325439,4.85745144448918));
#14732=CARTESIAN_POINT('Ctrl Pts',(-7.12604182038968,-3.99601069408371,
4.90487277263035));
#14733=CARTESIAN_POINT('Ctrl Pts',(-7.04819184769871,-4.40634676177701,
4.96169841481296));
#14734=CARTESIAN_POINT('Ctrl Pts',(-6.82636338655034,-4.7595056581786,5.01843153953646));
#14735=CARTESIAN_POINT('Ctrl Pts',(-6.49141297662963,-5.00640905746698,
5.07505897358501));
#14736=CARTESIAN_POINT('Ctrl Pts',(-6.09003751265709,-5.11411564108699,
5.13157085139478));
#14737=CARTESIAN_POINT('Ctrl Pts',(-5.6786123610455,-5.06726795065735,5.18795255071755));
#14738=CARTESIAN_POINT('Ctrl Pts',(-5.19017784555553,-4.81065089568624,
5.26294089870735));
#14739=CARTESIAN_POINT('Ctrl Pts',(-4.82877811722237,-4.18554821878284,
5.35628168565881));
#14740=CARTESIAN_POINT('Ctrl Pts',(-5.02211102820349,-3.34365258048631,
5.46759164112498));
#14741=CARTESIAN_POINT('Ctrl Pts',(-5.61197730680856,-2.94404370121664,
5.55969246505222));
#14742=CARTESIAN_POINT('Ctrl Pts',(-6.15048906815939,-2.9259067483885,5.63294612810208));
#14743=CARTESIAN_POINT('Ctrl Pts',(-6.57218830606153,-3.07274578152562,
5.69374353314818));
#14744=CARTESIAN_POINT('Ctrl Pts',(-6.92709063454883,-3.41928769105856,
5.76029112976678));
#14745=CARTESIAN_POINT('Ctrl Pts',(-7.08489845709846,-3.93331978001971,
5.83246177305221));
#14746=CARTESIAN_POINT('Ctrl Pts',(-6.97874255257226,-4.45701817474228,
5.90419082425952));
#14747=CARTESIAN_POINT('Ctrl Pts',(-6.6370356483897,-4.86355317377098,5.97546640233217));
#14748=CARTESIAN_POINT('Ctrl Pts',(-6.14579379656497,-5.05583391995401,
6.04627654027298));
#14749=CARTESIAN_POINT('Ctrl Pts',(-5.66925806099251,-4.99574215938401,
6.11075463056163));
#14750=CARTESIAN_POINT('Ctrl Pts',(-5.30691358174171,-4.76738235557255,
6.16902301258706));
#14751=CARTESIAN_POINT('Ctrl Pts',(-5.07930374249635,-4.45896349323313,
6.22119003887878));
#14752=CARTESIAN_POINT('Ctrl Pts',(-4.98082787805456,-4.09041784989305,
6.27308969220691));
#14753=CARTESIAN_POINT('Ctrl Pts',(-5.02349370691767,-3.71343965346201,
6.32471516558109));
#14754=CARTESIAN_POINT('Ctrl Pts',(-5.19999589872533,-3.37988542205928,
6.37606954207135));
#14755=CARTESIAN_POINT('Ctrl Pts',(-5.4847190912962,-3.13506427885037,6.42715348187171));
#14756=CARTESIAN_POINT('Ctrl Pts',(-5.83712621660341,-3.0121129912794,6.47796762234093));
#14757=CARTESIAN_POINT('Ctrl Pts',(-6.27051160587467,-3.0279850218392,6.5369435841435));
#14758=CARTESIAN_POINT('Ctrl Pts',(-6.71024506901487,-3.27130871222068,
6.60389475094362));
#14759=CARTESIAN_POINT('Ctrl Pts',(-6.98152291497359,-3.76371935754976,
6.67866321017483));
#14760=CARTESIAN_POINT('Ctrl Pts',(-6.95486940879079,-4.22678212803274,
6.74048184962521));
#14761=CARTESIAN_POINT('Ctrl Pts',(-6.78948845599291,-4.54563000849764,
6.78967337641285));
#14762=CARTESIAN_POINT('Ctrl Pts',(-6.58510503627771,-4.76139122419511,
6.8305173230869));
#14763=CARTESIAN_POINT('Ctrl Pts',(-6.18838065951204,-4.9729390553884,6.89153120571427));
#14764=CARTESIAN_POINT('Ctrl Pts',(-5.62852018163667,-4.92995885771748,
6.96424197979925));
#14765=CARTESIAN_POINT('Ctrl Pts',(-5.17930783991499,-4.52600430891302,
7.04445740123371));
#14766=CARTESIAN_POINT('Ctrl Pts',(-5.03049950675028,-4.00877291192731,
7.11621441643227));
#14767=CARTESIAN_POINT('Ctrl Pts',(-5.17961059739332,-3.49350571771481,
7.18758887136104));
#14768=CARTESIAN_POINT('Ctrl Pts',(-5.5773967358305,-3.13848926372906,7.25859618540072));
#14769=CARTESIAN_POINT('Ctrl Pts',(-6.10099673495183,-3.04979857717247,
7.32929304288679));
#14770=CARTESIAN_POINT('Ctrl Pts',(-6.58960034264882,-3.25249531366017,
7.39971414359334));
#14771=CARTESIAN_POINT('Ctrl Pts',(-6.89439488886565,-3.68259555007305,
7.46990161363075));
#14772=CARTESIAN_POINT('Ctrl Pts',(-6.92396663908848,-4.20760343729457,
7.53990591827929));
#14773=CARTESIAN_POINT('Ctrl Pts',(-6.66987225902436,-4.66687625782422,
7.60978068427827));
#14774=CARTESIAN_POINT('Ctrl Pts',(-6.21120047280729,-4.92032117302824,
7.67955308981974));
#14775=CARTESIAN_POINT('Ctrl Pts',(-5.68827856526509,-4.89095372189668,
7.74927925590553));
#14776=CARTESIAN_POINT('Ctrl Pts',(-5.26116058145738,-4.58792216788294,
7.81900282194838));
#14777=CARTESIAN_POINT('Ctrl Pts',(-5.0605146593326,-4.10382413158063,7.88877252132617));
#14778=CARTESIAN_POINT('Ctrl Pts',(-5.14832880834495,-3.58641746420325,
7.95863563783962));
#14779=CARTESIAN_POINT('Ctrl Pts',(-5.4984805112338,-3.19437254567264,8.02863688255444));
#14780=CARTESIAN_POINT('Ctrl Pts',(-6.0052116702054,-3.04798055828712,8.0988270789877));
#14781=CARTESIAN_POINT('Ctrl Pts',(-6.42855758612144,-3.16989299743707,
8.157498520417));
#14782=CARTESIAN_POINT('Ctrl Pts',(-6.69060506939908,-3.39192119413063,
8.20457536102132));
#14783=CARTESIAN_POINT('Ctrl Pts',(-6.87145241436045,-3.66176710955656,
8.24912648972436));
#14784=CARTESIAN_POINT('Ctrl Pts',(-6.9514390685762,-4.05527304704089,8.3030252977758));
#14785=CARTESIAN_POINT('Ctrl Pts',(-6.81226797661705,-4.50642896669386,
8.36639194934761));
#14786=CARTESIAN_POINT('Ctrl Pts',(-6.50137930109524,-4.81024489059206,
8.42475645360788));
#14787=CARTESIAN_POINT('Ctrl Pts',(-6.13147656542686,-4.93949375675132,
8.47805505000841));
#14788=CARTESIAN_POINT('Ctrl Pts',(-5.77783068564499,-4.92652168690223,
8.52621767484705));
#14789=CARTESIAN_POINT('Ctrl Pts',(-5.45197894534714,-4.78441519364883,
8.57458210426088));
#14790=CARTESIAN_POINT('Ctrl Pts',(-5.19943128109014,-4.53209841719623,
8.62316022836638));
#14791=CARTESIAN_POINT('Ctrl Pts',(-5.05584618525974,-4.20342880803269,
8.67195949129532));
#14792=CARTESIAN_POINT('Ctrl Pts',(-5.0422195366231,-3.84336351760004,8.72098742963023));
#14793=CARTESIAN_POINT('Ctrl Pts',(-5.16161137131951,-3.50154334879679,
8.77025177567099));
#14794=CARTESIAN_POINT('Ctrl Pts',(-5.39880490887244,-3.22561437898706,
8.81975828650979));
#14795=CARTESIAN_POINT('Ctrl Pts',(-5.72207914137123,-3.0546917552152,8.86951421619689));
#14796=CARTESIAN_POINT('Ctrl Pts',(-6.0872826786708,-3.01323072582504,8.91952319375617));
#14797=CARTESIAN_POINT('Ctrl Pts',(-6.444171507933,-3.10879395998011,8.96979185738356));
#14798=CARTESIAN_POINT('Ctrl Pts',(-6.74316713391831,-3.32908221727823,
9.02032286064399));
#14799=CARTESIAN_POINT('Ctrl Pts',(-6.94195230903849,-3.64511372710529,
9.07112086549811));
#14800=CARTESIAN_POINT('Ctrl Pts',(-7.01188601899995,-4.01392043220011,
9.12218639739436));
#14801=CARTESIAN_POINT('Ctrl Pts',(-6.94188943238603,-4.38461275011884,
9.17352468267902));
#14802=CARTESIAN_POINT('Ctrl Pts',(-6.71796764795472,-4.74180761880858,
9.23086676189624));
#14803=CARTESIAN_POINT('Ctrl Pts',(-6.32116660117755,-4.99875906667686,
9.29433422971609));
#14804=CARTESIAN_POINT('Ctrl Pts',(-5.80312100835904,-5.03811965025314,
9.36405136146833));
#14805=CARTESIAN_POINT('Ctrl Pts',(-5.30620047712063,-4.81454497903491,
9.43716931975444));
#14806=CARTESIAN_POINT('Ctrl Pts',(-4.97256942281115,-4.34579120199984,
9.5137592164803));
#14807=CARTESIAN_POINT('Ctrl Pts',(-4.93824840557943,-3.74461517188174,
9.59388490173077));
#14808=CARTESIAN_POINT('Ctrl Pts',(-5.23101010346705,-3.21365234345909,
9.67458646502851));
#14809=CARTESIAN_POINT('Ctrl Pts',(-5.76512274029881,-2.91777353632368,
9.75584554845314));
#14810=CARTESIAN_POINT('Ctrl Pts',(-6.37878312558969,-2.95168218807001,
9.83764095651353));
#14811=CARTESIAN_POINT('Ctrl Pts',(-6.88347692466996,-3.30911988689978,
9.91994818811354));
#14812=CARTESIAN_POINT('Ctrl Pts',(-7.12200435419038,-3.88366471751155,
10.0027398139742));
#14813=CARTESIAN_POINT('Ctrl Pts',(-7.01769174064254,-4.50040748652788,
10.0859855046625));
#14814=CARTESIAN_POINT('Ctrl Pts',(-6.5991026993888,-4.96945704213636,10.169652290447));
#14815=CARTESIAN_POINT('Ctrl Pts',(-5.99232847824897,-5.1446733592202,10.2537046806626));
#14816=CARTESIAN_POINT('Ctrl Pts',(-5.38283617149629,-4.96944471106765,
10.3381049457805));
#14817=CARTESIAN_POINT('Ctrl Pts',(-4.95848481508745,-4.49504806095511,
10.4228131773276));
#14818=CARTESIAN_POINT('Ctrl Pts',(-4.8512788133084,-3.86561185150167,10.5077878601832));
#14819=CARTESIAN_POINT('Ctrl Pts',(-5.09608303885727,-3.27408372793879,
10.5929853993213));
#14820=CARTESIAN_POINT('Ctrl Pts',(-5.61918598804022,-2.90272072154196,
10.6783618529632));
#14821=CARTESIAN_POINT('Ctrl Pts',(-6.26073803477781,-2.86658451987938,
10.7638698864798));
#14822=CARTESIAN_POINT('Ctrl Pts',(-6.82364327171669,-3.17764136170321,
10.8494663844497));
#14823=CARTESIAN_POINT('Ctrl Pts',(-7.13510597544169,-3.74083024574666,
10.9350962162971));
#14824=CARTESIAN_POINT('Ctrl Pts',(-7.09866726626603,-4.38320012653105,
11.0207290118911));
#14825=CARTESIAN_POINT('Ctrl Pts',(-6.72669125253576,-4.90762068704384,
11.1063111389501));
#14826=CARTESIAN_POINT('Ctrl Pts',(-6.13326093944664,-5.15321134684636,
11.1917885105552));
#14827=CARTESIAN_POINT('Ctrl Pts',(-5.5013182622223,-5.04585546444371,11.2771193767864));
#14828=CARTESIAN_POINT('Ctrl Pts',(-5.02452852733205,-4.61907390049617,
11.3622555821127));
#14829=CARTESIAN_POINT('Ctrl Pts',(-4.90711056796053,-4.21115651674335,
11.418857178779));
#14830=CARTESIAN_POINT('Ctrl Pts',(-4.90708301903907,-4.00651587433727,
11.447108175978));
#14831=CARTESIAN_POINT('Ctrl Pts',(-5.08958607327854,-3.99025782069458,
2.62934359726276));
#14832=CARTESIAN_POINT('Ctrl Pts',(-5.08960914627408,-3.81886565729437,
2.65300458397722));
#14833=CARTESIAN_POINT('Ctrl Pts',(-5.18775153299826,-3.47775231609314,
2.7003346517846));
#14834=CARTESIAN_POINT('Ctrl Pts',(-5.58803684598741,-3.11888353323257,
2.7718727663756));
#14835=CARTESIAN_POINT('Ctrl Pts',(-6.12129671315563,-3.02800055422244,
2.84387347131519));
#14836=CARTESIAN_POINT('Ctrl Pts',(-6.62498248189243,-3.23595716996215,
2.91641667550846));
#14837=CARTESIAN_POINT('Ctrl Pts',(-6.94329777941309,-3.68358881678574,
2.98951223929353));
#14838=CARTESIAN_POINT('Ctrl Pts',(-6.97483521943357,-4.23620018431934,
3.06319720344227));
#14839=CARTESIAN_POINT('Ctrl Pts',(-6.70566884665487,-4.72517502848787,
3.1374886735177));
#14840=CARTESIAN_POINT('Ctrl Pts',(-6.21320237967697,-4.99797593923465,
3.21240612526695));
#14841=CARTESIAN_POINT('Ctrl Pts',(-5.64636519782345,-4.96685768166421,
3.2879709618681));
#14842=CARTESIAN_POINT('Ctrl Pts',(-5.17888022725475,-4.6360306218548,3.36419310338532));
#14843=CARTESIAN_POINT('Ctrl Pts',(-4.95716603405221,-4.10260937681186,
3.44108212136025));
#14844=CARTESIAN_POINT('Ctrl Pts',(-5.05405766973863,-3.52801963757597,
3.51864211602294));
#14845=CARTESIAN_POINT('Ctrl Pts',(-5.44517562575364,-3.08929222903721,
3.5968739500623));
#14846=CARTESIAN_POINT('Ctrl Pts',(-6.01455473415458,-2.92453883772137,
3.67577419882147));
#14847=CARTESIAN_POINT('Ctrl Pts',(-6.58914066161724,-3.08930935334757,
3.75533567052421));
#14848=CARTESIAN_POINT('Ctrl Pts',(-6.97620465280587,-3.52165786554518,
3.83257632941237));
#14849=CARTESIAN_POINT('Ctrl Pts',(-7.06897925767441,-3.98066369790426,
3.89542955206584));
#14850=CARTESIAN_POINT('Ctrl Pts',(-7.01555893785241,-4.28254638624748,
3.93754537488261));
#14851=CARTESIAN_POINT('Ctrl Pts',(-6.95380842309345,-4.44582557552005,
3.96167160920718));
#14852=CARTESIAN_POINT('Ctrl Pts',(-6.83138672806294,-4.67780803645936,
3.99792061909243));
#14853=CARTESIAN_POINT('Ctrl Pts',(-6.5405370816015,-4.96217677817398,4.05251763409128));
#14854=CARTESIAN_POINT('Ctrl Pts',(-6.01531361240091,-5.11036494912871,
4.12576710362128));
#14855=CARTESIAN_POINT('Ctrl Pts',(-5.4798800948455,-4.98866772052924,4.19945314026379));
#14856=CARTESIAN_POINT('Ctrl Pts',(-5.10054865270113,-4.65370030513798,
4.26738027014));
#14857=CARTESIAN_POINT('Ctrl Pts',(-4.91834401520502,-4.2357863815548,4.32941472283313));
#14858=CARTESIAN_POINT('Ctrl Pts',(-4.90256885516074,-3.82420304826326,
4.38545643863725));
#14859=CARTESIAN_POINT('Ctrl Pts',(-5.03918037927126,-3.43420539707711,
4.44169518681064));
#14860=CARTESIAN_POINT('Ctrl Pts',(-5.33930525072368,-3.08446885471147,
4.50439031777555));
#14861=CARTESIAN_POINT('Ctrl Pts',(-5.80913211214926,-2.87223115930889,
4.57360189356491));
#14862=CARTESIAN_POINT('Ctrl Pts',(-6.37229427413888,-2.91422476933027,
4.64938345030258));
#14863=CARTESIAN_POINT('Ctrl Pts',(-6.74888177129849,-3.15750352412239,
4.709582128297));
#14864=CARTESIAN_POINT('Ctrl Pts',(-6.94490140998246,-3.41339882099762,
4.75401894510768));
#14865=CARTESIAN_POINT('Ctrl Pts',(-7.06970558341153,-3.66017127708851,
4.79214595145499));
#14866=CARTESIAN_POINT('Ctrl Pts',(-7.13500723247069,-4.00480166501556,
4.83987187277834));
#14867=CARTESIAN_POINT('Ctrl Pts',(-7.05655517105359,-4.41899249863413,
4.89723555158439));
#14868=CARTESIAN_POINT('Ctrl Pts',(-6.83208424000845,-4.77657076660703,
4.95467781113089));
#14869=CARTESIAN_POINT('Ctrl Pts',(-6.49207156199412,-5.02736404071781,
5.0121827474206));
#14870=CARTESIAN_POINT('Ctrl Pts',(-6.08339025242798,-5.13715599402453,
5.06973475823005));
#14871=CARTESIAN_POINT('Ctrl Pts',(-5.66322179904519,-5.08942531962948,
5.12731904881901));
#14872=CARTESIAN_POINT('Ctrl Pts',(-5.16297094376659,-4.82679185368301,
5.2041196620197));
#14873=CARTESIAN_POINT('Ctrl Pts',(-4.79066213150166,-4.18431414464998,
5.3001343861563));
#14874=CARTESIAN_POINT('Ctrl Pts',(-4.98965381173811,-3.31366183574818,
5.4152322895872));
#14875=CARTESIAN_POINT('Ctrl Pts',(-5.60225840489793,-2.89783757391139,
5.51095527979351));
#14876=CARTESIAN_POINT('Ctrl Pts',(-6.16385669310836,-2.87878317991021,
5.58735141171596));
#14877=CARTESIAN_POINT('Ctrl Pts',(-6.60462995607195,-3.03216488094667,
5.65090073233228));
#14878=CARTESIAN_POINT('Ctrl Pts',(-6.97665349261024,-3.39515151898213,
5.72063857301452));
#14879=CARTESIAN_POINT('Ctrl Pts',(-7.14265993135726,-3.93521632088349,
5.79647782910357));
#14880=CARTESIAN_POINT('Ctrl Pts',(-7.0310083056303,-4.4869108207016,5.87203948693374));
#14881=CARTESIAN_POINT('Ctrl Pts',(-6.67033948104626,-4.91626585048744,
5.94730014972142));
#14882=CARTESIAN_POINT('Ctrl Pts',(-6.15060695231922,-5.11985532484333,
6.02222597416855));
#14883=CARTESIAN_POINT('Ctrl Pts',(-5.64541150540802,-5.05627265809946,
6.09058083970922));
#14884=CARTESIAN_POINT('Ctrl Pts',(-5.26069476946472,-4.81388570953019,
6.15244175228014));
#14885=CARTESIAN_POINT('Ctrl Pts',(-5.01875583364388,-4.4861215358841,6.20788483808207));
#14886=CARTESIAN_POINT('Ctrl Pts',(-4.9139522084251,-4.09406610320522,6.26309574236783));
#14887=CARTESIAN_POINT('Ctrl Pts',(-4.95934334049254,-3.69270060694395,
6.31805861073807));
#14888=CARTESIAN_POINT('Ctrl Pts',(-5.14735742783483,-3.33732783794384,
6.37276806703712));
#14889=CARTESIAN_POINT('Ctrl Pts',(-5.45082896178906,-3.07635399284825,
6.42721536466454));
#14890=CARTESIAN_POINT('Ctrl Pts',(-5.82657935181436,-2.94524248695214,
6.48139347544157));
#14891=CARTESIAN_POINT('Ctrl Pts',(-6.28875793296553,-2.96214980134559,
6.54428133364918));
#14892=CARTESIAN_POINT('Ctrl Pts',(-6.7577138250312,-3.221654892675,6.61568080479831));
#14893=CARTESIAN_POINT('Ctrl Pts',(-7.046869499807,-3.74657137930345,6.69536653730686));
#14894=CARTESIAN_POINT('Ctrl Pts',(-7.01842122365346,-4.23984048730701,
6.76121511684626));
#14895=CARTESIAN_POINT('Ctrl Pts',(-6.84239266572927,-4.57917463164239,
6.81356230981021));
#14896=CARTESIAN_POINT('Ctrl Pts',(-6.62501763362136,-4.8086423485827,6.85699845424774));
#14897=CARTESIAN_POINT('Ctrl Pts',(-6.20340460181096,-5.03340444241976,
6.921826051713));
#14898=CARTESIAN_POINT('Ctrl Pts',(-5.60959457936301,-4.98752605922673,
6.99894677554392));
#14899=CARTESIAN_POINT('Ctrl Pts',(-5.13461428204011,-4.56008255639909,
7.08377299672669));
#14900=CARTESIAN_POINT('Ctrl Pts',(-4.9778500212962,-4.01441171084717,7.15945663213478));
#14901=CARTESIAN_POINT('Ctrl Pts',(-5.13490417096659,-3.4726580148424,7.23449301164271));
#14902=CARTESIAN_POINT('Ctrl Pts',(-5.55195715900246,-3.10081935662606,
7.30889700246225));
#14903=CARTESIAN_POINT('Ctrl Pts',(-6.09863068969014,-3.00854209579386,
7.3826886113079));
#14904=CARTESIAN_POINT('Ctrl Pts',(-6.60648447138017,-3.21958594141858,
7.45589041854474));
#14905=CARTESIAN_POINT('Ctrl Pts',(-6.9216791982701,-3.66497931973675,7.52852965123266));
#14906=CARTESIAN_POINT('Ctrl Pts',(-6.95177924004462,-4.20587447720696,
7.60063489875532));
#14907=CARTESIAN_POINT('Ctrl Pts',(-6.6909662386489,-4.67646854269574,7.67223803710999));
#14908=CARTESIAN_POINT('Ctrl Pts',(-6.22299726037103,-4.93459747092674,
7.7433777926895));
#14909=CARTESIAN_POINT('Ctrl Pts',(-5.69254032107038,-4.90439315263447,
7.81409150036152));
#14910=CARTESIAN_POINT('Ctrl Pts',(-5.2618365955028,-4.59831452234616,7.88442076722058));
#14911=CARTESIAN_POINT('Ctrl Pts',(-5.06089011399604,-4.11241503492589,
7.95440897609695));
#14912=CARTESIAN_POINT('Ctrl Pts',(-5.14891476057707,-3.5962099799928,8.02410112276677));
#14913=CARTESIAN_POINT('Ctrl Pts',(-5.49666377882435,-3.20746270201702,
8.09354551735423));
#14914=CARTESIAN_POINT('Ctrl Pts',(-5.99681265084705,-3.06340348104051,
8.16278786553222));
#14915=CARTESIAN_POINT('Ctrl Pts',(-6.41224590200003,-3.18336826033736,
8.22037117887724));
#14916=CARTESIAN_POINT('Ctrl Pts',(-6.66836775683141,-3.40046253258805,
8.26638619207942));
#14917=CARTESIAN_POINT('Ctrl Pts',(-6.84466758932173,-3.66362380044245,
8.30982365803551));
#14918=CARTESIAN_POINT('Ctrl Pts',(-6.92216235674791,-4.04596600254198,
8.36217057302082));
#14919=CARTESIAN_POINT('Ctrl Pts',(-6.78729405069043,-4.48230953614279,
8.42346277729895));
#14920=CARTESIAN_POINT('Ctrl Pts',(-6.48766998582839,-4.77482452426569,
8.47967703069394));
#14921=CARTESIAN_POINT('Ctrl Pts',(-6.13255927907409,-4.8987822245107,8.53083176826075));
#14922=CARTESIAN_POINT('Ctrl Pts',(-5.79405373663887,-4.88627598976337,
8.57692529241349));
#14923=CARTESIAN_POINT('Ctrl Pts',(-5.48301690867117,-4.7505320540268,8.62309299030759));
#14924=CARTESIAN_POINT('Ctrl Pts',(-5.24260511121906,-4.51022473960559,
8.6693420733107));
#14925=CARTESIAN_POINT('Ctrl Pts',(-5.10628760740664,-4.19799093789299,
8.71569057208715));
#14926=CARTESIAN_POINT('Ctrl Pts',(-5.09344745751731,-3.85672818834445,
8.76215292714239));
#14927=CARTESIAN_POINT('Ctrl Pts',(-5.2064383924313,-3.53345566112826,8.80874199058791));
#14928=CARTESIAN_POINT('Ctrl Pts',(-5.43040665899872,-3.27300345792075,
8.85547704096572));
#14929=CARTESIAN_POINT('Ctrl Pts',(-5.73509299001327,-3.11197616335786,
8.90236484872161));
#14930=CARTESIAN_POINT('Ctrl Pts',(-6.07874463617352,-3.07301201788798,
8.94941993516621));
#14931=CARTESIAN_POINT('Ctrl Pts',(-6.41409907073854,-3.16285967160041,
8.9966547034903));
#14932=CARTESIAN_POINT('Ctrl Pts',(-6.69471463191465,-3.36965539654581,
9.04408229994015));
#14933=CARTESIAN_POINT('Ctrl Pts',(-6.88108384841174,-3.66601330952044,
9.09171381385298));
#14934=CARTESIAN_POINT('Ctrl Pts',(-6.9465780164732,-4.01156860735228,9.13955827692911));
#14935=CARTESIAN_POINT('Ctrl Pts',(-6.88101508718794,-4.35867292221011,
9.18763006950063));
#14936=CARTESIAN_POINT('Ctrl Pts',(-6.67141125514706,-4.6929894095024,9.24130109606731));
#14937=CARTESIAN_POINT('Ctrl Pts',(-6.30010945166128,-4.93341342253205,
9.300689301377));
#14938=CARTESIAN_POINT('Ctrl Pts',(-5.81536145282493,-4.97024504354847,
9.36592731075453));
#14939=CARTESIAN_POINT('Ctrl Pts',(-5.35021909987976,-4.76099072350817,
9.43437195900332));
#14940=CARTESIAN_POINT('Ctrl Pts',(-5.03767451365318,-4.32196228839712,
9.50611541884564));
#14941=CARTESIAN_POINT('Ctrl Pts',(-5.00539919271839,-3.7582617467778,9.58125324423978));
#14942=CARTESIAN_POINT('Ctrl Pts',(-5.28020380225241,-3.25961343195422,
9.65704139684407));
#14943=CARTESIAN_POINT('Ctrl Pts',(-5.78257562978636,-2.98114555664001,
9.73349075256426));
#14944=CARTESIAN_POINT('Ctrl Pts',(-6.36108530515163,-3.012933580896,9.81060861195967));
#14945=CARTESIAN_POINT('Ctrl Pts',(-6.83813479497314,-3.35054278443211,
9.8883982005671));
#14946=CARTESIAN_POINT('Ctrl Pts',(-7.06436526891603,-3.89486967330545,
9.9668588526319));
#14947=CARTESIAN_POINT('Ctrl Pts',(-6.9654778242667,-4.48105551001564,10.0459859100048));
#14948=CARTESIAN_POINT('Ctrl Pts',(-6.5665776770944,-4.92845750971493,10.1257707953368));
#14949=CARTESIAN_POINT('Ctrl Pts',(-5.9861285159527,-5.09638198019228,10.2062010449906));
#14950=CARTESIAN_POINT('Ctrl Pts',(-5.40077430176762,-4.92842380855109,
10.2872603721036));
#14951=CARTESIAN_POINT('Ctrl Pts',(-4.99147369823858,-4.47135751604514,
10.3689288026212));
#14952=CARTESIAN_POINT('Ctrl Pts',(-4.88737185959524,-3.86224827783339,
10.4511826978566));
#14953=CARTESIAN_POINT('Ctrl Pts',(-5.12493606869768,-3.2872555983534,10.5339951511892));
#14954=CARTESIAN_POINT('Ctrl Pts',(-5.6352408565221,-2.92451464581263,10.6173355355939));
#14955=CARTESIAN_POINT('Ctrl Pts',(-6.2640751739065,-2.88870996291299,10.7011710889467));
#14956=CARTESIAN_POINT('Ctrl Pts',(-6.81848291382748,-3.19462273696641,
10.7854640234358));
#14957=CARTESIAN_POINT('Ctrl Pts',(-7.12686484968034,-3.75143580561001,
10.870178671056));
#14958=CARTESIAN_POINT('Ctrl Pts',(-7.09106689040093,-4.38964946962175,
10.9552663097424));
#14959=CARTESIAN_POINT('Ctrl Pts',(-6.72015560018353,-4.91323638810909,
11.0406886438574));
#14960=CARTESIAN_POINT('Ctrl Pts',(-6.12535013441635,-5.15984551571332,
11.1263955783573));
#14961=CARTESIAN_POINT('Ctrl Pts',(-5.4888177159,-5.05207984615036,11.2123531394243));
#14962=CARTESIAN_POINT('Ctrl Pts',(-5.00618128684596,-4.62072035504479,
11.2984791152375));
#14963=CARTESIAN_POINT('Ctrl Pts',(-4.88655223846457,-4.20611915635318,
11.3560320854752));
#14964=CARTESIAN_POINT('Ctrl Pts',(-4.88652420961371,-3.9979134719832,11.3847752429281));
#14965=CARTESIAN_POINT('Ctrl Pts',(-5.11146388820137,-4.00349311292524,
2.72519423144341));
#14966=CARTESIAN_POINT('Ctrl Pts',(-5.1114863896228,-3.83634674945349,2.74826907808176));
#14967=CARTESIAN_POINT('Ctrl Pts',(-5.2073386709242,-3.50459135808253,2.79432654428865));
#14968=CARTESIAN_POINT('Ctrl Pts',(-5.59392162451954,-3.15886603128654,
2.86334120921819));
#14969=CARTESIAN_POINT('Ctrl Pts',(-6.10462882761145,-3.07233116043825,
2.93229890548955));
#14970=CARTESIAN_POINT('Ctrl Pts',(-6.58324742293624,-3.27049009618399,
3.00126508671495));
#14971=CARTESIAN_POINT('Ctrl Pts',(-6.88338780506893,-3.69336482148996,
3.07028562510752));
#14972=CARTESIAN_POINT('Ctrl Pts',(-6.9125378234219,-4.21176138753265,3.13941249417303));
#14973=CARTESIAN_POINT('Ctrl Pts',(-6.66117842543386,-4.66753315377219,
3.20869846013298));
#14974=CARTESIAN_POINT('Ctrl Pts',(-6.20426035603016,-4.92022504844555,
3.27819713364705));
#14975=CARTESIAN_POINT('Ctrl Pts',(-5.68113059624983,-4.89117330402607,
3.34794822940351));
#14976=CARTESIAN_POINT('Ctrl Pts',(-5.25170796397958,-4.58692564876463,
3.41800289998785));
#14977=CARTESIAN_POINT('Ctrl Pts',(-5.04895699031254,-4.09847602344442,
3.48840459466937));
#14978=CARTESIAN_POINT('Ctrl Pts',(-5.13758843731787,-3.57411477941281,
3.5591972982065));
#14979=CARTESIAN_POINT('Ctrl Pts',(-5.49375906320309,-3.17483235058257,
3.63042148845005));
#14980=CARTESIAN_POINT('Ctrl Pts',(-6.01112620351243,-3.02524985044883,
3.7021155619589));
#14981=CARTESIAN_POINT('Ctrl Pts',(-6.53249037329618,-3.17483138875088,
3.77431501475635));
#14982=CARTESIAN_POINT('Ctrl Pts',(-6.88345308070225,-3.56688559200541,
3.84435825865076));
#14983=CARTESIAN_POINT('Ctrl Pts',(-6.96758670253936,-3.98305434767195,
3.90134832783096));
#14984=CARTESIAN_POINT('Ctrl Pts',(-6.91914662613188,-4.25684126103168,
3.93954468754766));
#14985=CARTESIAN_POINT('Ctrl Pts',(-6.86313250970625,-4.40495668933761,
3.96143027230283));
#14986=CARTESIAN_POINT('Ctrl Pts',(-6.75206286997603,-4.61543115327382,
3.99431845667718));
#14987=CARTESIAN_POINT('Ctrl Pts',(-6.48808491278166,-4.8736085272702,4.04387852104861));
#14988=CARTESIAN_POINT('Ctrl Pts',(-6.01074296926441,-5.00838471988809,
4.11045312998563));
#14989=CARTESIAN_POINT('Ctrl Pts',(-5.52325638980643,-4.89771417726584,
4.17753632489081));
#14990=CARTESIAN_POINT('Ctrl Pts',(-5.17709404353748,-4.59222957518482,
4.23950256233906));
#14991=CARTESIAN_POINT('Ctrl Pts',(-5.01043388242926,-4.21016874273666,
4.29621843833516));
#14992=CARTESIAN_POINT('Ctrl Pts',(-4.99589713399363,-3.83310074843265,
4.34755840879351));
#14993=CARTESIAN_POINT('Ctrl Pts',(-5.12125994677539,-3.47495912195723,
4.39919681737111));
#14994=CARTESIAN_POINT('Ctrl Pts',(-5.39743127754854,-3.15296659074283,
4.45690341966157));
#14995=CARTESIAN_POINT('Ctrl Pts',(-5.83115129685322,-2.95679680521155,
4.52080615558924));
#14996=CARTESIAN_POINT('Ctrl Pts',(-6.35316218281195,-2.99545324585569,
4.5910453945408));
#14997=CARTESIAN_POINT('Ctrl Pts',(-6.70376257092702,-3.22166688646999,
4.64705710233426));
#14998=CARTESIAN_POINT('Ctrl Pts',(-6.88678372913165,-3.46054900968793,
4.68853934391483));
#14999=CARTESIAN_POINT('Ctrl Pts',(-7.0035074423105,-3.69129846575723,4.72419072967401));
#15000=CARTESIAN_POINT('Ctrl Pts',(-7.06484203667896,-4.01438157828431,
4.76893210034011));
#15001=CARTESIAN_POINT('Ctrl Pts',(-6.99115886817154,-4.40411780678025,
4.82290082050557));
#15002=CARTESIAN_POINT('Ctrl Pts',(-6.77930308964722,-4.74188330839879,
4.87714191961237));
#15003=CARTESIAN_POINT('Ctrl Pts',(-6.45705491738398,-4.97974523614269,
4.93165021696835));
#15004=CARTESIAN_POINT('Ctrl Pts',(-6.06815028839713,-5.08439258892097,
4.98641872200361));
#15005=CARTESIAN_POINT('Ctrl Pts',(-5.66662034905994,-5.03892039260337,
5.04143952880628));
#15006=CARTESIAN_POINT('Ctrl Pts',(-5.18655285081867,-4.78714708110153,
5.11512653518091));
#15007=CARTESIAN_POINT('Ctrl Pts',(-4.82613499448797,-4.16740651020841,
5.20781216493432));
#15008=CARTESIAN_POINT('Ctrl Pts',(-5.01848603257964,-3.31910069175158,
5.31989761553554));
#15009=CARTESIAN_POINT('Ctrl Pts',(-5.61981332624524,-2.9094932624567,5.41393698760798));
#15010=CARTESIAN_POINT('Ctrl Pts',(-6.17547145334383,-2.89038655816394,
5.48950913679716));
#15011=CARTESIAN_POINT('Ctrl Pts',(-6.61354799505512,-3.04263063984369,
5.55265712784929));
#15012=CARTESIAN_POINT('Ctrl Pts',(-6.98549988101616,-3.40498346435387,
5.62232050138183));
#15013=CARTESIAN_POINT('Ctrl Pts',(-7.15276763293528,-3.94768190565954,
5.69853201897246));
#15014=CARTESIAN_POINT('Ctrl Pts',(-7.04028187626715,-4.50564202791614,
5.77493404150203));
#15015=CARTESIAN_POINT('Ctrl Pts',(-6.67370872730767,-4.94268691087855,
5.8514836989803));
#15016=CARTESIAN_POINT('Ctrl Pts',(-6.14199125879717,-5.15141832358651,
5.92815184332714));
#15017=CARTESIAN_POINT('Ctrl Pts',(-5.62193267759359,-5.08634477712989,
5.99850052868461));
#15018=CARTESIAN_POINT('Ctrl Pts',(-5.22382985790438,-4.83573996048168,
6.06248404381697));
#15019=CARTESIAN_POINT('Ctrl Pts',(-4.97233041446878,-4.49530252943299,
6.12008460662565));
#15020=CARTESIAN_POINT('Ctrl Pts',(-4.86283729649089,-4.08632133851381,
6.17767307025924));
#15021=CARTESIAN_POINT('Ctrl Pts',(-4.91023011228302,-3.66584228236825,
6.2352433234891));
#15022=CARTESIAN_POINT('Ctrl Pts',(-5.10784440922835,-3.29200270232238,
6.29277619099215));
#15023=CARTESIAN_POINT('Ctrl Pts',(-5.42817465514537,-3.01632843786686,
6.35025789696987));
#15024=CARTESIAN_POINT('Ctrl Pts',(-5.82638908712853,-2.87723611583061,
6.40767362354461));
#15025=CARTESIAN_POINT('Ctrl Pts',(-6.31803709458161,-2.89504436194142,
6.47456205294508));
#15026=CARTESIAN_POINT('Ctrl Pts',(-6.81932677366183,-3.17198486831857,
6.55085313024292));
#15027=CARTESIAN_POINT('Ctrl Pts',(-7.13022853870334,-3.73544410660141,
6.63640199512977));
#15028=CARTESIAN_POINT('Ctrl Pts',(-7.09985484999904,-4.26766588322049,
6.70744516442597));
#15029=CARTESIAN_POINT('Ctrl Pts',(-6.90937626959466,-4.63499910749687,
6.7640986891494));
#15030=CARTESIAN_POINT('Ctrl Pts',(-6.67363197611175,-4.88389416051919,
6.81120623918702));
#15031=CARTESIAN_POINT('Ctrl Pts',(-6.21540678092779,-5.1283578591014,6.88167501898689));
#15032=CARTESIAN_POINT('Ctrl Pts',(-5.56750905972414,-5.07878760962261,
6.96581377607078));
#15033=CARTESIAN_POINT('Ctrl Pts',(-5.04725897731621,-4.61100994769211,
7.05867824449733));
#15034=CARTESIAN_POINT('Ctrl Pts',(-4.87502236930835,-4.01211284223512,
7.14174757031646));
#15035=CARTESIAN_POINT('Ctrl Pts',(-5.04762190701414,-3.41622257144757,
7.22427184785083));
#15036=CARTESIAN_POINT('Ctrl Pts',(-5.50694650780015,-3.00656473703432,
7.3062269716042));
#15037=CARTESIAN_POINT('Ctrl Pts',(-6.10967519422246,-2.90477651653003,
7.38758405539665));
#15038=CARTESIAN_POINT('Ctrl Pts',(-6.66982264240046,-3.13755152778926,
7.46832293040742));
#15039=CARTESIAN_POINT('Ctrl Pts',(-7.01735971004567,-3.62873051387297,
7.54842470644817));
#15040=CARTESIAN_POINT('Ctrl Pts',(-7.05042704618396,-4.22472296521213,
7.62787559478529));
#15041=CARTESIAN_POINT('Ctrl Pts',(-6.76331769359956,-4.74244592149819,
7.70666504495723));
#15042=CARTESIAN_POINT('Ctrl Pts',(-6.24935597182185,-5.02571530571555,
7.78478624180885));
#15043=CARTESIAN_POINT('Ctrl Pts',(-5.66841983881672,-4.992387139032,7.86223669086622));
#15044=CARTESIAN_POINT('Ctrl Pts',(-5.19841826828567,-4.65801741457885,
7.93901781676939));
#15045=CARTESIAN_POINT('Ctrl Pts',(-4.98021276748805,-4.12948856160228,
8.0151347855238));
#15046=CARTESIAN_POINT('Ctrl Pts',(-5.07589799354624,-3.57067831525686,
8.09059738471413));
#15047=CARTESIAN_POINT('Ctrl Pts',(-5.45083661313803,-3.1521641999378,8.1654177239109));
#15048=CARTESIAN_POINT('Ctrl Pts',(-5.98682154391905,-2.99827751934189,
8.23961543820677));
#15049=CARTESIAN_POINT('Ctrl Pts',(-6.42909049947727,-3.12640964775913,
8.30093785873061));
#15050=CARTESIAN_POINT('Ctrl Pts',(-6.70043358144534,-3.35653176806574,
8.3497078062489));
#15051=CARTESIAN_POINT('Ctrl Pts',(-6.88657968867636,-3.63453023876189,
8.39558817150443));
#15052=CARTESIAN_POINT('Ctrl Pts',(-6.96771103676148,-4.03652906886562,
8.45063175096959));
#15053=CARTESIAN_POINT('Ctrl Pts',(-6.82648710559109,-4.49210420145525,
8.51464865041861));
#15054=CARTESIAN_POINT('Ctrl Pts',(-6.51539277681862,-4.79529496351186,
8.57297461574563));
#15055=CARTESIAN_POINT('Ctrl Pts',(-6.14916965403812,-4.92292264363337,
8.62573226691127));
#15056=CARTESIAN_POINT('Ctrl Pts',(-5.80196913848439,-4.909917389324,8.67302067136497));
#15057=CARTESIAN_POINT('Ctrl Pts',(-5.48474830529899,-4.77128250666151,
8.72012180414365));
#15058=CARTESIAN_POINT('Ctrl Pts',(-5.24095336372299,-4.52733379926624,
8.76705651381845));
#15059=CARTESIAN_POINT('Ctrl Pts',(-5.10357198259525,-4.21220488751096,
8.81383360157659));
#15060=CARTESIAN_POINT('Ctrl Pts',(-5.09086860733029,-3.8697568592241,8.86046614728715));
#15061=CARTESIAN_POINT('Ctrl Pts',(-5.20379231374995,-3.54721450725183,
8.90696898921786));
#15062=CARTESIAN_POINT('Ctrl Pts',(-5.42617914586712,-3.28888235937374,
8.95334950953911));
#15063=CARTESIAN_POINT('Ctrl Pts',(-5.72694661343973,-3.13011803590362,
8.99962946343878));
#15064=CARTESIAN_POINT('Ctrl Pts',(-6.06427021742266,-3.09205710176064,
9.04582166245532));
#15065=CARTESIAN_POINT('Ctrl Pts',(-6.39160236864643,-3.17992456672212,
9.09194056693847));
#15066=CARTESIAN_POINT('Ctrl Pts',(-6.66398918720521,-3.38086998734912,
9.13799988910989));
#15067=CARTESIAN_POINT('Ctrl Pts',(-6.84387671595628,-3.66722063438552,
9.18401494103932));
#15068=CARTESIAN_POINT('Ctrl Pts',(-6.9066670679967,-3.9993466547744,9.23000347197484));
#15069=CARTESIAN_POINT('Ctrl Pts',(-6.84382580193358,-4.33123468360912,
9.27597545458883));
#15070=CARTESIAN_POINT('Ctrl Pts',(-6.64420674116633,-4.6493173671815,9.32706132906817));
#15071=CARTESIAN_POINT('Ctrl Pts',(-6.29259770566886,-4.87662537775517,
9.38327712956274));
#15072=CARTESIAN_POINT('Ctrl Pts',(-5.83643195943725,-4.91096143644274,
9.44467383294874));
#15073=CARTESIAN_POINT('Ctrl Pts',(-5.40126345522019,-4.71485427181151,
9.50873917863421));
#15074=CARTESIAN_POINT('Ctrl Pts',(-5.11067191095492,-4.3060141160397,9.57552502373875));
#15075=CARTESIAN_POINT('Ctrl Pts',(-5.08114749160738,-3.78409491879455,
9.64510336845023));
#15076=CARTESIAN_POINT('Ctrl Pts',(-5.33465759113435,-3.32474188581643,
9.71495303907397));
#15077=CARTESIAN_POINT('Ctrl Pts',(-5.79582326317987,-3.06943273025373,
9.78512080947981));
#15078=CARTESIAN_POINT('Ctrl Pts',(-6.32483990648236,-3.09873681028405,
9.85565111386688));
#15079=CARTESIAN_POINT('Ctrl Pts',(-6.75970042212355,-3.40672284706517,
9.92658636274972));
#15080=CARTESIAN_POINT('Ctrl Pts',(-6.96536307562826,-3.90194183503021,
9.99796648875838));
#15081=CARTESIAN_POINT('Ctrl Pts',(-6.87546272288741,-4.43425542219748,
10.0698288137258));
#15082=CARTESIAN_POINT('Ctrl Pts',(-6.51357040107586,-4.84006961009873,
10.1422077693513));
#15083=CARTESIAN_POINT('Ctrl Pts',(-5.987291243916,-4.99231483046356,10.215134731367));
#15084=CARTESIAN_POINT('Ctrl Pts',(-5.45650767309877,-4.84005420013297,
10.2886378275285));
#15085=CARTESIAN_POINT('Ctrl Pts',(-5.08506221166951,-4.42538406867581,
10.3627417782245));
#15086=CARTESIAN_POINT('Ctrl Pts',(-4.990363336042,-3.87204197816745,10.4374677368732));
#15087=CARTESIAN_POINT('Ctrl Pts',(-5.20641176001674,-3.34868167362847,
10.5128331669689));
#15088=CARTESIAN_POINT('Ctrl Pts',(-5.67177590318358,-3.01762544047152,
10.5888517859959));
#15089=CARTESIAN_POINT('Ctrl Pts',(-6.24696780354825,-2.98461711370722,
10.6655333487327));
#15090=CARTESIAN_POINT('Ctrl Pts',(-6.75588576872762,-3.26509285809973,
10.7428838921771));
#15091=CARTESIAN_POINT('Ctrl Pts',(-7.04023081280776,-3.777787551644,10.8209050268513));
#15092=CARTESIAN_POINT('Ctrl Pts',(-7.00749304795215,-4.36808121544397,
10.8995954448141));
#15093=CARTESIAN_POINT('Ctrl Pts',(-6.66323831848384,-4.85473674137387,
10.9789522846304));
#15094=CARTESIAN_POINT('Ctrl Pts',(-6.10814274891664,-5.08536413962976,
11.0589563184805));
#15095=CARTESIAN_POINT('Ctrl Pts',(-5.51078426858185,-4.98467662470909,
11.1396132151697));
#15096=CARTESIAN_POINT('Ctrl Pts',(-5.05510117731205,-4.57809092709479,
11.2208625878388));
#15097=CARTESIAN_POINT('Ctrl Pts',(-4.94130014896063,-4.18467098041075,
11.275481957862));
#15098=CARTESIAN_POINT('Ctrl Pts',(-4.94127348351102,-3.98659299949179,
11.3028269682096));
#15099=CARTESIAN_POINT('Ctrl Pts',(-5.04970734608444,-4.014134093399,2.80233410707682));
#15100=CARTESIAN_POINT('Ctrl Pts',(-5.04973134605583,-3.83585611419469,
2.82694569265781));
#15101=CARTESIAN_POINT('Ctrl Pts',(-5.15206923445116,-3.4823776986807,2.8760204246601));
#15102=CARTESIAN_POINT('Ctrl Pts',(-5.5614206316956,-3.1170823820106,2.9490162429901));
#15103=CARTESIAN_POINT('Ctrl Pts',(-6.09810765925963,-3.02662690392752,
3.02147152025646));
#15104=CARTESIAN_POINT('Ctrl Pts',(-6.59712262306125,-3.23386828229798,
3.09339820603842));
#15105=CARTESIAN_POINT('Ctrl Pts',(-6.90732475729933,-3.67194259316541,
3.1648380955771));
#15106=CARTESIAN_POINT('Ctrl Pts',(-6.93665430754779,-4.20438646265423,
3.23582612292702));
#15107=CARTESIAN_POINT('Ctrl Pts',(-6.68004065809059,-4.6684075873074,3.30640045570415));
#15108=CARTESIAN_POINT('Ctrl Pts',(-6.21810008921364,-4.92314954604884,
3.37659939052329));
#15109=CARTESIAN_POINT('Ctrl Pts',(-5.69397648524808,-4.8934201192585,3.4464749107676));
#15110=CARTESIAN_POINT('Ctrl Pts',(-5.26764630093375,-4.59059929678225,
3.51606935423513));
#15111=CARTESIAN_POINT('Ctrl Pts',(-5.06841388342893,-4.10903719737237,
3.58543200219124));
#15112=CARTESIAN_POINT('Ctrl Pts',(-5.15562823873306,-3.59663109925005,
3.65461124945938));
#15113=CARTESIAN_POINT('Ctrl Pts',(-5.50139878391617,-3.20987562699863,
3.72365749828155));
#15114=CARTESIAN_POINT('Ctrl Pts',(-5.99930358470049,-3.0664980755698,3.79262171549619));
#15115=CARTESIAN_POINT('Ctrl Pts',(-6.49701819772681,-3.20984963236153,
3.86155496989464));
#15116=CARTESIAN_POINT('Ctrl Pts',(-6.82941314564483,-3.58189551733825,
3.92795571781378));
#15117=CARTESIAN_POINT('Ctrl Pts',(-6.90838988314061,-3.97403261720178,
3.98163963232954));
#15118=CARTESIAN_POINT('Ctrl Pts',(-6.86289779162592,-4.23089029905683,
4.01747350728414));
#15119=CARTESIAN_POINT('Ctrl Pts',(-6.81044462585338,-4.36957346598223,
4.03796496216898));
#15120=CARTESIAN_POINT('Ctrl Pts',(-6.70657469009075,-4.56638426544445,
4.06871708209625));
#15121=CARTESIAN_POINT('Ctrl Pts',(-6.46041372675795,-4.80683684920928,
4.11489392405871));
#15122=CARTESIAN_POINT('Ctrl Pts',(-6.01759168782143,-4.93159391025523,
4.17664209312006));
#15123=CARTESIAN_POINT('Ctrl Pts',(-5.56748440020554,-4.82915336507103,
4.23858440378004));
#15124=CARTESIAN_POINT('Ctrl Pts',(-5.24923420310336,-4.54803781304708,
4.29557297658576));
#15125=CARTESIAN_POINT('Ctrl Pts',(-5.09649486695971,-4.19765775733976,
4.34757880141343));
#15126=CARTESIAN_POINT('Ctrl Pts',(-5.08327146603833,-3.8527045728546,4.39454228313687));
#15127=CARTESIAN_POINT('Ctrl Pts',(-5.19778067898822,-3.5257764501926,4.4416810635407));
#15128=CARTESIAN_POINT('Ctrl Pts',(-5.44949654344042,-3.23240173071767,
4.49426376054938));
#15129=CARTESIAN_POINT('Ctrl Pts',(-5.84405907648008,-3.05405527712975,
4.5523889489519));
#15130=CARTESIAN_POINT('Ctrl Pts',(-6.31813331118975,-3.0892458106026,4.61617835220101));
#15131=CARTESIAN_POINT('Ctrl Pts',(-6.63615534979497,-3.2945021411286,4.66698598908312));
#15132=CARTESIAN_POINT('Ctrl Pts',(-6.80211652576663,-3.51112312284911,
4.70460183160974));
#15133=CARTESIAN_POINT('Ctrl Pts',(-6.90794042502969,-3.72033578077783,
4.73692473637605));
#15134=CARTESIAN_POINT('Ctrl Pts',(-6.96353651155719,-4.01321756900286,
4.77748340064075));
#15135=CARTESIAN_POINT('Ctrl Pts',(-6.8967395362674,-4.36654451491255,4.82640965537421));
#15136=CARTESIAN_POINT('Ctrl Pts',(-6.70462301696789,-4.67285941150863,
4.87559975444018));
#15137=CARTESIAN_POINT('Ctrl Pts',(-6.41222708309043,-4.88870995426925,
4.9250602957143));
#15138=CARTESIAN_POINT('Ctrl Pts',(-6.05905690187772,-4.98377296921959,
4.97479876152583));
#15139=CARTESIAN_POINT('Ctrl Pts',(-5.69401310371,-4.94246805059484,5.02481952450994));
#15140=CARTESIAN_POINT('Ctrl Pts',(-5.25700058678662,-4.71334498855493,
5.09189738429313));
#15141=CARTESIAN_POINT('Ctrl Pts',(-4.92782438010502,-4.14811605570046,
5.17646870468282));
#15142=CARTESIAN_POINT('Ctrl Pts',(-5.10336010603255,-3.37095253982733,
5.27914266109507));
#15143=CARTESIAN_POINT('Ctrl Pts',(-5.65645834162634,-2.99345132990119,
5.36570023443787));
#15144=CARTESIAN_POINT('Ctrl Pts',(-6.1699913664732,-2.97563873503376,5.43554293217881));
#15145=CARTESIAN_POINT('Ctrl Pts',(-6.57603542854649,-3.11664200174749,
5.49407461937123));
#15146=CARTESIAN_POINT('Ctrl Pts',(-6.92218952721961,-3.4535052357566,5.55887865709695));
#15147=CARTESIAN_POINT('Ctrl Pts',(-7.07875034877777,-3.96045691179561,
5.63008959061315));
#15148=CARTESIAN_POINT('Ctrl Pts',(-6.97347642065377,-4.48421269602345,
5.70180458156708));
#15149=CARTESIAN_POINT('Ctrl Pts',(-6.62798627215935,-4.89664122684824,
5.774012746944));
#15150=CARTESIAN_POINT('Ctrl Pts',(-6.12405454097509,-5.09484079360517,
5.84669765808443));
#15151=CARTESIAN_POINT('Ctrl Pts',(-5.62839476656752,-5.03315023883122,
5.91374936242762));
#15152=CARTESIAN_POINT('Ctrl Pts',(-5.24707290574412,-4.79332552679213,
5.97502813879928));
#15153=CARTESIAN_POINT('Ctrl Pts',(-5.00513094556786,-4.46608144539262,
6.0304158049875));
#15154=CARTESIAN_POINT('Ctrl Pts',(-4.89923307934873,-4.07118717667332,
6.08603667815864));
#15155=CARTESIAN_POINT('Ctrl Pts',(-4.94503254732023,-3.66338243335723,
6.14187603551199));
#15156=CARTESIAN_POINT('Ctrl Pts',(-5.13737019634667,-3.2991604706762,6.19792514865836));
#15157=CARTESIAN_POINT('Ctrl Pts',(-5.45065975015127,-3.02931466187735,
6.25417235306358));
#15158=CARTESIAN_POINT('Ctrl Pts',(-5.84195458942871,-2.89246212692768,
6.31060529244871));
#15159=CARTESIAN_POINT('Ctrl Pts',(-6.32729017217876,-2.90982944532215,
6.37664874935649));
#15160=CARTESIAN_POINT('Ctrl Pts',(-6.82518249543237,-3.18428897290923,
6.45238921757374));
#15161=CARTESIAN_POINT('Ctrl Pts',(-7.13653729570471,-3.74723934336787,
6.53793129879579));
#15162=CARTESIAN_POINT('Ctrl Pts',(-7.10645173764727,-4.28288462039874,
6.60943086415581));
#15163=CARTESIAN_POINT('Ctrl Pts',(-6.91387636050383,-4.65453678643226,
6.66674636099218));
#15164=CARTESIAN_POINT('Ctrl Pts',(-6.67463855570598,-4.90719225117517,
6.7145634081676));
#15165=CARTESIAN_POINT('Ctrl Pts',(-6.20793365325718,-5.15650233906366,
6.78637308174185));
#15166=CARTESIAN_POINT('Ctrl Pts',(-5.54326866993286,-5.10667068723003,
6.8726820373125));
#15167=CARTESIAN_POINT('Ctrl Pts',(-5.00498017679516,-4.62367347193851,
6.96868726861754));
#15168=CARTESIAN_POINT('Ctrl Pts',(-4.82528676773444,-4.00081830567214,
7.05510807363504));
#15169=CARTESIAN_POINT('Ctrl Pts',(-5.0053951436861,-3.37689823861283,7.14150364401192));
#15170=CARTESIAN_POINT('Ctrl Pts',(-5.48872482401552,-2.94511360670821,
7.22781068048454));
#15171=CARTESIAN_POINT('Ctrl Pts',(-6.12700755803508,-2.83678576185677,
7.31398732955836));
#15172=CARTESIAN_POINT('Ctrl Pts',(-6.72375384707874,-3.08423079176768,
7.3999797427674));
#15173=CARTESIAN_POINT('Ctrl Pts',(-7.09619313569336,-3.60980021306789,
7.48573840517752));
#15174=CARTESIAN_POINT('Ctrl Pts',(-7.13220207582214,-4.25095033753033,
7.57121852214645));
#15175=CARTESIAN_POINT('Ctrl Pts',(-6.82226807006467,-4.8106779703119,7.65637806859443));
#15176=CARTESIAN_POINT('Ctrl Pts',(-6.26467177253605,-5.11841193742535,
7.74116325228304));
#15177=CARTESIAN_POINT('Ctrl Pts',(-5.6318275183675,-5.08243517581132,7.82553668780451));
#15178=CARTESIAN_POINT('Ctrl Pts',(-5.11797960895723,-4.71721968706553,
7.90945703925193));
#15179=CARTESIAN_POINT('Ctrl Pts',(-4.87859187879085,-4.13801197139399,
7.99288822687277));
#15180=CARTESIAN_POINT('Ctrl Pts',(-4.98352628418032,-3.52404020081029,
8.07579636929506));
#15181=CARTESIAN_POINT('Ctrl Pts',(-5.39610472469272,-3.06329341970928,
8.15814987354169));
#15182=CARTESIAN_POINT('Ctrl Pts',(-5.98679900925825,-2.89359357100788,
8.23992344671619));
#15183=CARTESIAN_POINT('Ctrl Pts',(-6.47460873131575,-3.03488339301435,
8.30755819903438));
#15184=CARTESIAN_POINT('Ctrl Pts',(-6.7739262603932,-3.2887285566142,8.361354258082));
#15185=CARTESIAN_POINT('Ctrl Pts',(-6.97925131350371,-3.59536714231701,
8.41196069057612));
#15186=CARTESIAN_POINT('Ctrl Pts',(-7.06869487572216,-4.03865184085066,
8.47265070023439));
#15187=CARTESIAN_POINT('Ctrl Pts',(-6.91302940167929,-4.5405717591675,8.54318103210321));
#15188=CARTESIAN_POINT('Ctrl Pts',(-6.57067014159411,-4.87411806202039,
8.60735327160586));
#15189=CARTESIAN_POINT('Ctrl Pts',(-6.16833388604433,-5.01426844190105,
8.66530637083758));
#15190=CARTESIAN_POINT('Ctrl Pts',(-5.78753541605273,-4.99995160631877,
8.71716535362411));
#15191=CARTESIAN_POINT('Ctrl Pts',(-5.44029859859097,-4.84812019841673,
8.76872529749127));
#15192=CARTESIAN_POINT('Ctrl Pts',(-5.17404859244767,-4.58160005133281,
8.81998703566189));
#15193=CARTESIAN_POINT('Ctrl Pts',(-5.02442632985894,-4.23818465699728,
8.87095201100959));
#15194=CARTESIAN_POINT('Ctrl Pts',(-5.01071327042434,-3.86603779547018,
8.92162223867994));
#15195=CARTESIAN_POINT('Ctrl Pts',(-5.133161597464,-3.51659961675723,8.97200070786022));
#15196=CARTESIAN_POINT('Ctrl Pts',(-5.37343817646623,-3.23765328783206,
9.02209162753279));
#15197=CARTESIAN_POINT('Ctrl Pts',(-5.69721379739349,-3.06688291613834,
9.07189898149531));
#15198=CARTESIAN_POINT('Ctrl Pts',(-6.05895785997844,-3.02618452117534,
9.12142738396272));
#15199=CARTESIAN_POINT('Ctrl Pts',(-6.40855782530253,-3.12017328225075,
9.1706837654698));
#15200=CARTESIAN_POINT('Ctrl Pts',(-6.69823038132667,-3.33403896702626,
9.21967431232278));
#15201=CARTESIAN_POINT('Ctrl Pts',(-6.88863293580495,-3.63740928685802,
9.26840700272366));
#15202=CARTESIAN_POINT('Ctrl Pts',(-6.95467920020127,-3.98761029148836,
9.3168884619293));
#15203=CARTESIAN_POINT('Ctrl Pts',(-6.88857999906526,-4.33587510882518,
9.365129823227));
#15204=CARTESIAN_POINT('Ctrl Pts',(-6.67995054872608,-4.66795372110108,
9.41847144777411));
#15205=CARTESIAN_POINT('Ctrl Pts',(-6.31469728103988,-4.9036483621764,9.47683205548445));
#15206=CARTESIAN_POINT('Ctrl Pts',(-5.84433052501836,-4.93863276025009,
9.54012573212548));
#15207=CARTESIAN_POINT('Ctrl Pts',(-5.39902615361661,-4.73746267851064,
9.6056963980877));
#15208=CARTESIAN_POINT('Ctrl Pts',(-5.10430163036973,-4.32178849006536,
9.67352801570003));
#15209=CARTESIAN_POINT('Ctrl Pts',(-5.075187070932,-3.79592840074772,9.74361293322054));
#15210=CARTESIAN_POINT('Ctrl Pts',(-5.32901434535869,-3.33728385728079,
9.81338743259124));
#15211=CARTESIAN_POINT('Ctrl Pts',(-5.78624334014352,-3.08485820545814,
9.88289796408472));
#15212=CARTESIAN_POINT('Ctrl Pts',(-6.30604928044245,-3.11425799421081,
9.95219289498374));
#15213=CARTESIAN_POINT('Ctrl Pts',(-6.72956367609471,-3.41493193430552,
10.021321716681));
#15214=CARTESIAN_POINT('Ctrl Pts',(-6.92790783320255,-3.89402420811448,
10.0903350063486));
#15215=CARTESIAN_POINT('Ctrl Pts',(-6.84109464889487,-4.40474031567081,
10.1592840124265));
#15216=CARTESIAN_POINT('Ctrl Pts',(-6.49597320364271,-4.79095463264426,
10.2282203670656));
#15217=CARTESIAN_POINT('Ctrl Pts',(-5.99800616609963,-4.93448878448542,
10.2971957723242));
#15218=CARTESIAN_POINT('Ctrl Pts',(-5.49933195557159,-4.79095105026251,
10.3662617164922));
#15219=CARTESIAN_POINT('Ctrl Pts',(-5.1527139367811,-4.40334569175967,10.4354691299253));
#15220=CARTESIAN_POINT('Ctrl Pts',(-5.06514889324528,-3.8893268520199,10.5048681455515));
#15221=CARTESIAN_POINT('Ctrl Pts',(-5.26513463485952,-3.40581804738845,
10.5745075879262));
#15222=CARTESIAN_POINT('Ctrl Pts',(-5.69343493256485,-3.10151979632748,
10.6444352547726));
#15223=CARTESIAN_POINT('Ctrl Pts',(-6.22052717215153,-3.07154871751346,
10.7146962814146));
#15224=CARTESIAN_POINT('Ctrl Pts',(-6.68521110233421,-3.32791229650645,
10.7853358376373));
#15225=CARTESIAN_POINT('Ctrl Pts',(-6.9440279852268,-3.7949758640772,10.8563922071995));
#15226=CARTESIAN_POINT('Ctrl Pts',(-6.91413085988338,-4.33148339801506,
10.927911347834));
#15227=CARTESIAN_POINT('Ctrl Pts',(-6.60162688016772,-4.77309716981846,
10.9999287290131));
#15228=CARTESIAN_POINT('Ctrl Pts',(-6.09828367789878,-4.9821600137055,11.0724702098908));
#15229=CARTESIAN_POINT('Ctrl Pts',(-5.55679798821165,-4.89091465998753,
11.1455776779411));
#15230=CARTESIAN_POINT('Ctrl Pts',(-5.14358275601793,-4.5222302433581,11.2192552432817));
#15231=CARTESIAN_POINT('Ctrl Pts',(-5.04025189628822,-4.16531630046125,
11.2688069686638));
#15232=CARTESIAN_POINT('Ctrl Pts',(-5.04022766416365,-3.9853136985979,11.2936566414427));
#15233=CARTESIAN_POINT('Ctrl Pts',(-4.95040444753908,-4.01407741549073,
2.80202038668682));
#15234=CARTESIAN_POINT('Ctrl Pts',(-4.95043088631308,-3.81768338133247,
2.82913292521151));
#15235=CARTESIAN_POINT('Ctrl Pts',(-5.06328046757572,-3.42769328904537,
2.88327944150245));
#15236=CARTESIAN_POINT('Ctrl Pts',(-5.51483986880678,-3.02481655682361,
2.96379357401038));
#15237=CARTESIAN_POINT('Ctrl Pts',(-6.10663155887047,-2.92510416783479,
3.04369524283156));
#15238=CARTESIAN_POINT('Ctrl Pts',(-6.65627932676067,-3.15350765201444,
3.12292801020133));
#15239=CARTESIAN_POINT('Ctrl Pts',(-6.9972996120088,-3.63538358706421,3.20150185546868));
#15240=CARTESIAN_POINT('Ctrl Pts',(-7.02927375427223,-4.21966673835877,
3.27940299578842));
#15241=CARTESIAN_POINT('Ctrl Pts',(-6.7482428987564,-4.72729484195001,3.35663488008679));
#15242=CARTESIAN_POINT('Ctrl Pts',(-6.24433772797396,-5.00482166130207,
3.43319919431017));
#15243=CARTESIAN_POINT('Ctrl Pts',(-5.67509809740256,-4.97217848865363,
3.50910146535417));
#15244=CARTESIAN_POINT('Ctrl Pts',(-5.21440956091332,-4.64446921121479,
3.58435286234765));
#15245=CARTESIAN_POINT('Ctrl Pts',(-5.00052648608049,-4.12635602119185,
3.65896760418264));
#15246=CARTESIAN_POINT('Ctrl Pts',(-5.09426410583311,-3.57844077526578,
3.73296399244798));
#15247=CARTESIAN_POINT('Ctrl Pts',(-5.46214956932136,-3.16771217138052,
3.80636392097382));
#15248=CARTESIAN_POINT('Ctrl Pts',(-5.98800389280316,-3.01684552839974,
3.87919268136819));
#15249=CARTESIAN_POINT('Ctrl Pts',(-6.50966711131542,-3.16768533912665,
3.95147944874766));
#15250=CARTESIAN_POINT('Ctrl Pts',(-6.85516841335202,-3.55524247398461,
4.02059719986475));
#15251=CARTESIAN_POINT('Ctrl Pts',(-6.93640504947824,-3.96044008918348,
4.07607464042623));
#15252=CARTESIAN_POINT('Ctrl Pts',(-6.88959590680744,-4.22437715215301,
4.11290351758767));
#15253=CARTESIAN_POINT('Ctrl Pts',(-6.83583101050569,-4.36650480320736,
4.13390569410839));
#15254=CARTESIAN_POINT('Ctrl Pts',(-6.7295526054213,-4.5678453422278,4.16536800412348));
#15255=CARTESIAN_POINT('Ctrl Pts',(-6.4785719176604,-4.81253370237805,4.21242247700862));
#15256=CARTESIAN_POINT('Ctrl Pts',(-6.03075890744692,-4.93824024016166,
4.27485498317197));
#15257=CARTESIAN_POINT('Ctrl Pts',(-5.57912503362765,-4.83500621126696,
4.33703045129724));
#15258=CARTESIAN_POINT('Ctrl Pts',(-5.26234982431842,-4.55465959483225,
4.39381979062297));
#15259=CARTESIAN_POINT('Ctrl Pts',(-5.11135697875295,-4.20781103939821,
4.44529674263384));
#15260=CARTESIAN_POINT('Ctrl Pts',(-5.09852187023819,-3.86824490814822,
4.49153434459407));
#15261=CARTESIAN_POINT('Ctrl Pts',(-5.21076926661952,-3.54825343245558,
4.53768901317022));
#15262=CARTESIAN_POINT('Ctrl Pts',(-5.4560334473407,-3.26270136286835,4.5888995411409));
#15263=CARTESIAN_POINT('Ctrl Pts',(-5.83799792334387,-3.09044094457653,
4.64515534859482));
#15264=CARTESIAN_POINT('Ctrl Pts',(-6.29359570267334,-3.12464990354928,
4.70646757272288));
#15265=CARTESIAN_POINT('Ctrl Pts',(-6.5971317711187,-3.32088855862012,4.75500854197238));
#15266=CARTESIAN_POINT('Ctrl Pts',(-6.75487078461784,-3.52682180277232,
4.79077023674625));
#15267=CARTESIAN_POINT('Ctrl Pts',(-6.85522021528563,-3.72525753530104,
4.82142962589092));
#15268=CARTESIAN_POINT('Ctrl Pts',(-6.90765078845783,-4.00210628009459,
4.85976988485919));
#15269=CARTESIAN_POINT('Ctrl Pts',(-6.84466700781614,-4.33458160329838,
4.90581898898127));
#15270=CARTESIAN_POINT('Ctrl Pts',(-6.66451131395465,-4.62157482642531,
4.95192414686361));
#15271=CARTESIAN_POINT('Ctrl Pts',(-6.39151660574891,-4.82296908084052,
4.99809965612829));
#15272=CARTESIAN_POINT('Ctrl Pts',(-6.06305555872298,-4.91125610532342,
5.04435858184245));
#15273=CARTESIAN_POINT('Ctrl Pts',(-5.72479607824289,-4.87288998099965,
5.09071672932403));
#15274=CARTESIAN_POINT('Ctrl Pts',(-5.32120053858948,-4.66111598189267,
5.15267699940499));
#15275=CARTESIAN_POINT('Ctrl Pts',(-5.01901830093614,-4.14106232858579,
5.2304571964414));
#15276=CARTESIAN_POINT('Ctrl Pts',(-5.18022338687198,-3.43017789857566,
5.32440560742871));
#15277=CARTESIAN_POINT('Ctrl Pts',(-5.6844669484819,-3.08645264353291,5.40329988483335));
#15278=CARTESIAN_POINT('Ctrl Pts',(-6.15144238874992,-3.07029944892001,
5.46681719664217));
#15279=CARTESIAN_POINT('Ctrl Pts',(-6.52026173698852,-3.19841233327777,
5.51998619154465));
#15280=CARTESIAN_POINT('Ctrl Pts',(-6.83432988576568,-3.50411755194789,
5.57879302796362));
#15281=CARTESIAN_POINT('Ctrl Pts',(-6.97628146059944,-3.96381837777065,
5.64337000548355));
#15282=CARTESIAN_POINT('Ctrl Pts',(-6.88084694300038,-4.43864700704047,
5.70838686985743));
#15283=CARTESIAN_POINT('Ctrl Pts',(-6.56758301987762,-4.81266288881362,
5.77386709056138));
#15284=CARTESIAN_POINT('Ctrl Pts',(-6.11031818471074,-4.99257534235218,
5.83982471574392));
#15285=CARTESIAN_POINT('Ctrl Pts',(-5.66001412277134,-4.93661451797503,
5.90073884439067));
#15286=CARTESIAN_POINT('Ctrl Pts',(-5.31308429830285,-4.71849225798761,
5.95648421056427));
#15287=CARTESIAN_POINT('Ctrl Pts',(-5.09263031894632,-4.42040358314247,
6.00694184124335));
#15288=CARTESIAN_POINT('Ctrl Pts',(-4.99593329451219,-4.06008832376263,
6.05769248289879));
#15289=CARTESIAN_POINT('Ctrl Pts',(-5.03772761005556,-3.68727382498282,
6.10873703661228));
#15290=CARTESIAN_POINT('Ctrl Pts',(-5.21384768597732,-3.35358843624591,
6.1600783267073));
#15291=CARTESIAN_POINT('Ctrl Pts',(-5.5014279300585,-3.10576378920885,6.21171698888381));
#15292=CARTESIAN_POINT('Ctrl Pts',(-5.86154480647318,-2.97971897775594,
6.26365397549107));
#15293=CARTESIAN_POINT('Ctrl Pts',(-6.30941327345328,-2.99561470365393,
6.32459355700482));
#15294=CARTESIAN_POINT('Ctrl Pts',(-6.77065800699938,-3.24951148750743,
6.39473524121105));
#15295=CARTESIAN_POINT('Ctrl Pts',(-7.0607018985248,-3.77301027291914,6.47429880651946));
#15296=CARTESIAN_POINT('Ctrl Pts',(-7.03292138795243,-4.27386006447141,
6.54114742255594));
#15297=CARTESIAN_POINT('Ctrl Pts',(-6.85223599948128,-4.62277890659896,
6.59494154091868));
#15298=CARTESIAN_POINT('Ctrl Pts',(-6.62708269893594,-4.86061413836101,
6.63994414492635));
#15299=CARTESIAN_POINT('Ctrl Pts',(-6.18654127549617,-5.09621068018119,
6.70774704639851));
#15300=CARTESIAN_POINT('Ctrl Pts',(-5.55521460528796,-5.04973111393953,
6.78971417043737));
#15301=CARTESIAN_POINT('Ctrl Pts',(-5.03992134796692,-4.5883040965929,6.88151516750169));
#15302=CARTESIAN_POINT('Ctrl Pts',(-4.86647072351276,-3.98899998152023,
6.96467750538145));
#15303=CARTESIAN_POINT('Ctrl Pts',(-5.04035634712671,-3.3845330871616,7.04834093198449));
#15304=CARTESIAN_POINT('Ctrl Pts',(-5.51120006351292,-2.96311388418359,
7.13247929982247));
#15305=CARTESIAN_POINT('Ctrl Pts',(-6.13755247913796,-2.85620971181115,
7.21704708882013));
#15306=CARTESIAN_POINT('Ctrl Pts',(-6.72743904042145,-3.10014807205115,
7.30200621015969));
#15307=CARTESIAN_POINT('Ctrl Pts',(-7.09845727328089,-3.62266975603267,
7.38731447687665));
#15308=CARTESIAN_POINT('Ctrl Pts',(-7.13514378651329,-4.26482661359482,
7.47292307371327));
#15309=CARTESIAN_POINT('Ctrl Pts',(-6.82312421498377,-4.82958152399516,
7.55878062096553));
#15310=CARTESIAN_POINT('Ctrl Pts',(-6.25727921934041,-5.14256327876596,
7.64484924170431));
#15311=CARTESIAN_POINT('Ctrl Pts',(-5.61038110386298,-5.10639049644132,
7.73107411010418));
#15312=CARTESIAN_POINT('Ctrl Pts',(-5.0813191910786,-4.73109282931615,7.81740648211959));
#15313=CARTESIAN_POINT('Ctrl Pts',(-4.83286177762465,-4.13147349319584,
7.90379432673586));
#15314=CARTESIAN_POINT('Ctrl Pts',(-4.94165930199982,-3.4914906721837,7.99018552170849));
#15315=CARTESIAN_POINT('Ctrl Pts',(-5.3738945619569,-3.00797620488942,8.07652992915658));
#15316=CARTESIAN_POINT('Ctrl Pts',(-5.99684003484179,-2.82845004799815,
8.1627717509804));
#15317=CARTESIAN_POINT('Ctrl Pts',(-6.51449684023436,-2.97795530901467,
8.23452455634887));
#15318=CARTESIAN_POINT('Ctrl Pts',(-6.83340937345703,-3.24831236496221,
8.29182387018181));
#15319=CARTESIAN_POINT('Ctrl Pts',(-7.05275944220763,-3.57577124194805,
8.3458718722718));
#15320=CARTESIAN_POINT('Ctrl Pts',(-7.14888836510883,-4.05081892701449,
8.41090607558749));
#15321=CARTESIAN_POINT('Ctrl Pts',(-6.98158887614932,-4.59121631424625,
8.48682539302922));
#15322=CARTESIAN_POINT('Ctrl Pts',(-6.6117457325826,-4.95188043527737,8.55617619977002));
#15323=CARTESIAN_POINT('Ctrl Pts',(-6.17552481242006,-5.10395058079544,
8.61900798734293));
#15324=CARTESIAN_POINT('Ctrl Pts',(-5.76155504078242,-5.08847730642841,
8.6753791908211));
#15325=CARTESIAN_POINT('Ctrl Pts',(-5.3831114419134,-4.92309348031777,8.73156508207711));
#15326=CARTESIAN_POINT('Ctrl Pts',(-5.09226942582765,-4.63206374041745,
8.78754752252364));
#15327=CARTESIAN_POINT('Ctrl Pts',(-4.92846639521676,-4.25626808792367,
8.84331833042908));
#15328=CARTESIAN_POINT('Ctrl Pts',(-4.91337499340381,-3.84826985979358,
8.89886725533888));
#15329=CARTESIAN_POINT('Ctrl Pts',(-5.04778839460805,-3.46454521355224,
8.95418338540694));
#15330=CARTESIAN_POINT('Ctrl Pts',(-5.31195836233809,-3.15779237445369,
9.00926172959177));
#15331=CARTESIAN_POINT('Ctrl Pts',(-5.66836068440024,-2.96977926794819,
9.06408851803747));
#15332=CARTESIAN_POINT('Ctrl Pts',(-6.0669191210522,-2.92491551484476,9.11865767650999));
#15333=CARTESIAN_POINT('Ctrl Pts',(-6.45235041531044,-3.02852547184126,
9.17296094526983));
#15334=CARTESIAN_POINT('Ctrl Pts',(-6.77183369988165,-3.26439524326313,
9.2269931450209));
#15335=CARTESIAN_POINT('Ctrl Pts',(-6.98185220328006,-3.59902874792769,
9.28074746802313));
#15336=CARTESIAN_POINT('Ctrl Pts',(-7.05467848322916,-3.98526890769635,
9.33421836644156));
#15337=CARTESIAN_POINT('Ctrl Pts',(-6.98178576790913,-4.36920823973671,
9.38740267928406));
#15338=CARTESIAN_POINT('Ctrl Pts',(-6.75190034469451,-4.73504959901346,
9.44617221538153));
#15339=CARTESIAN_POINT('Ctrl Pts',(-6.34988721691645,-4.99435744148628,
9.51039990537655));
#15340=CARTESIAN_POINT('Ctrl Pts',(-5.833124943149,-5.03265791293926,9.57993884000276));
#15341=CARTESIAN_POINT('Ctrl Pts',(-5.34505445198339,-4.81197730828659,
9.6518236665488));
#15342=CARTESIAN_POINT('Ctrl Pts',(-5.02312104102536,-4.35746827773343,
9.72597446942884));
#15343=CARTESIAN_POINT('Ctrl Pts',(-4.99173885665344,-3.78474783904724,
9.80231093424411));
#15344=CARTESIAN_POINT('Ctrl Pts',(-5.26733037366742,-3.28753608995048,
9.87798912154192));
#15345=CARTESIAN_POINT('Ctrl Pts',(-5.7610100142267,-3.01545532543433,9.95302085463951));
#15346=CARTESIAN_POINT('Ctrl Pts',(-6.31901312620276,-3.04746542801833,
10.0274218227863));
#15347=CARTESIAN_POINT('Ctrl Pts',(-6.77073258958868,-3.36875755220951,
10.1012114179017));
#15348=CARTESIAN_POINT('Ctrl Pts',(-6.98060223215716,-3.87703875799955,
10.1744126613645));
#15349=CARTESIAN_POINT('Ctrl Pts',(-6.88862190599467,-4.41490833473546,
10.2470520646821));
#15350=CARTESIAN_POINT('Ctrl Pts',(-6.52726603979659,-4.81843912722608,
10.3191594492329));
#15351=CARTESIAN_POINT('Ctrl Pts',(-6.01022364648023,-4.96686190627768,
10.390767804212));
#15352=CARTESIAN_POINT('Ctrl Pts',(-5.49680133015996,-4.81845446474053,
10.4619130490713));
#15353=CARTESIAN_POINT('Ctrl Pts',(-5.14312970083041,-4.42204619402635,
10.5326339259449));
#15354=CARTESIAN_POINT('Ctrl Pts',(-5.05500684830352,-3.90108130763402,
10.6029715447986));
#15355=CARTESIAN_POINT('Ctrl Pts',(-5.25654917398459,-3.41542914409823,
10.6729696033374));
#15356=CARTESIAN_POINT('Ctrl Pts',(-5.68373908537632,-3.11267812572593,
10.7426732040747));
#15357=CARTESIAN_POINT('Ctrl Pts',(-6.20470547300614,-3.08367627152615,
10.8121306435434));
#15358=CARTESIAN_POINT('Ctrl Pts',(-6.6599080173046,-3.33549556127491,10.8813885520368));
#15359=CARTESIAN_POINT('Ctrl Pts',(-6.91104727221352,-3.78995831176175,
10.9505019065133));
#15360=CARTESIAN_POINT('Ctrl Pts',(-6.88163942109489,-4.30749866343159,
11.0195109771094));
#15361=CARTESIAN_POINT('Ctrl Pts',(-6.58197977005813,-4.73002117605488,
11.0884704057876));
#15362=CARTESIAN_POINT('Ctrl Pts',(-6.10331498315377,-4.92825339378842,
11.157438247149));
#15363=CARTESIAN_POINT('Ctrl Pts',(-5.59217136013618,-4.84169576209836,
11.2264590988613));
#15364=CARTESIAN_POINT('Ctrl Pts',(-5.20484579854406,-4.49541939104753,
11.2955951659005));
#15365=CARTESIAN_POINT('Ctrl Pts',(-5.10870499490301,-4.16277367149241,
11.3417785121125));
#15366=CARTESIAN_POINT('Ctrl Pts',(-5.10868242823946,-3.99514255262147,
11.3649202801113));
#15367=CARTESIAN_POINT('Ctrl Pts',(-4.88818719635698,-4.00347727294065,
2.72529722008525));
#15368=CARTESIAN_POINT('Ctrl Pts',(-4.8882151797164,-3.79560965978366,2.75399370617715));
#15369=CARTESIAN_POINT('Ctrl Pts',(-5.00768402952602,-3.38176479254249,
2.8114458207661));
#15370=CARTESIAN_POINT('Ctrl Pts',(-5.48912761258474,-2.95155104882261,
2.89735388716427));
#15371=CARTESIAN_POINT('Ctrl Pts',(-6.12367588859993,-2.84418536850341,
2.9830394830188));
#15372=CARTESIAN_POINT('Ctrl Pts',(-6.71608295773462,-3.08988004512223,
3.06841689939367));
#15373=CARTESIAN_POINT('Ctrl Pts',(-7.08548551208247,-3.61116247844501,
3.15345759772618));
#15374=CARTESIAN_POINT('Ctrl Pts',(-7.12058610325535,-4.24603336903534,
3.23810936636211));
#15375=CARTESIAN_POINT('Ctrl Pts',(-6.81439089049297,-4.79977673821013,
3.32233710953462));
#15376=CARTESIAN_POINT('Ctrl Pts',(-6.26324852083861,-5.10364407717512,
3.40610338036098));
#15377=CARTESIAN_POINT('Ctrl Pts',(-5.63880259300186,-5.06806358715257,
3.489365903903));
#15378=CARTESIAN_POINT('Ctrl Pts',(-5.1322299275751,-4.70793906273771,3.57209477752228));
#15379=CARTESIAN_POINT('Ctrl Pts',(-4.89657596527452,-4.13743625505341,
3.65425891220947));
#15380=CARTESIAN_POINT('Ctrl Pts',(-4.99983412380025,-3.53336895261622,
3.73583244193299));
#15381=CARTESIAN_POINT('Ctrl Pts',(-5.4056138863883,-3.08027815183281,3.81679205719959));
#15382=CARTESIAN_POINT('Ctrl Pts',(-5.98566419848572,-2.9138752058618,3.89711855437139));
#15383=CARTESIAN_POINT('Ctrl Pts',(-6.5607175758941,-3.08021552425877,3.97679599518704));
#15384=CARTESIAN_POINT('Ctrl Pts',(-6.94104043806148,-3.50699914121927,
4.05288638067068));
#15385=CARTESIAN_POINT('Ctrl Pts',(-7.03023256912709,-3.95237226486497,
4.11385241520314));
#15386=CARTESIAN_POINT('Ctrl Pts',(-6.97884494814435,-4.24201642458273,
4.15426575236254));
#15387=CARTESIAN_POINT('Ctrl Pts',(-6.91989134069545,-4.39785579457805,
4.17729322914019));
#15388=CARTESIAN_POINT('Ctrl Pts',(-6.80342892392235,-4.61848748240129,
4.21176796422099));
#15389=CARTESIAN_POINT('Ctrl Pts',(-6.52880823922492,-4.88607101119092,
4.2632233953033));
#15390=CARTESIAN_POINT('Ctrl Pts',(-6.040337156624,-5.02298743966762,4.33131125112158));
#15391=CARTESIAN_POINT('Ctrl Pts',(-5.54956390280064,-4.91056640618497,
4.39887183410603));
#15392=CARTESIAN_POINT('Ctrl Pts',(-5.20684987950378,-4.60696587191263,
4.46032308612493));
#15393=CARTESIAN_POINT('Ctrl Pts',(-5.04416577721804,-4.23292269389065,
4.51582356884532));
#15394=CARTESIAN_POINT('Ctrl Pts',(-5.03048913212015,-3.86809303813757,
4.56548891208506));
#15395=CARTESIAN_POINT('Ctrl Pts',(-5.15075591711637,-3.52565244918924,
4.61488073233877));
#15396=CARTESIAN_POINT('Ctrl Pts',(-5.41232829565927,-3.22134006592063,
4.66945984212975));
#15397=CARTESIAN_POINT('Ctrl Pts',(-5.81764466923774,-3.03889776937362,
4.72912569596472));
#15398=CARTESIAN_POINT('Ctrl Pts',(-6.29802642946598,-3.07534304184591,
4.79377063220834));
#15399=CARTESIAN_POINT('Ctrl Pts',(-6.61583128941994,-3.28116081870527,
4.84458999703416));
#15400=CARTESIAN_POINT('Ctrl Pts',(-6.78033519526549,-3.49597871671357,
4.88188763378668));
#15401=CARTESIAN_POINT('Ctrl Pts',(-6.88472108499998,-3.70245984060303,
4.91378208472349));
#15402=CARTESIAN_POINT('Ctrl Pts',(-6.93893227813884,-3.98943532436169,
4.9535135694603));
#15403=CARTESIAN_POINT('Ctrl Pts',(-6.87381560608202,-4.33220427041261,
5.00098425193981));
#15404=CARTESIAN_POINT('Ctrl Pts',(-6.68890774242002,-4.62645671922366,
5.04825821317051));
#15405=CARTESIAN_POINT('Ctrl Pts',(-6.41032716352109,-4.83174064470429,
5.09534896646907));
#15406=CARTESIAN_POINT('Ctrl Pts',(-6.07704473350618,-4.92113376655074,
5.14227039283988));
#15407=CARTESIAN_POINT('Ctrl Pts',(-5.73578768023823,-4.88225536268528,
5.1890341934005));
#15408=CARTESIAN_POINT('Ctrl Pts',(-5.33090189374131,-4.66950551714918,
5.25119580619967));
#15409=CARTESIAN_POINT('Ctrl Pts',(-5.03127344889024,-4.15143713732072,
5.32855279023866));
#15410=CARTESIAN_POINT('Ctrl Pts',(-5.19141108346178,-3.45225578202365,
5.42097872761472));
#15411=CARTESIAN_POINT('Ctrl Pts',(-5.68285225510471,-3.11865945660659,
5.49774652619562));
#15412=CARTESIAN_POINT('Ctrl Pts',(-6.13381349440763,-3.10330694154298,
5.55908224617128));
#15413=CARTESIAN_POINT('Ctrl Pts',(-6.48818012667083,-3.22657080017143,
5.61016324701949));
#15414=CARTESIAN_POINT('Ctrl Pts',(-6.78797228127654,-3.51887282825301,
5.66633206213167));
#15415=CARTESIAN_POINT('Ctrl Pts',(-6.92236393580735,-3.95532434325643,
5.72761512040668));
#15416=CARTESIAN_POINT('Ctrl Pts',(-6.83198717655826,-4.40328470381393,
5.78895467537118));
#15417=CARTESIAN_POINT('Ctrl Pts',(-6.53784519235893,-4.75395986679681,
5.85037529513985));
#15418=CARTESIAN_POINT('Ctrl Pts',(-6.11102395408416,-4.92157115925373,
5.91192019317696));
#15419=CARTESIAN_POINT('Ctrl Pts',(-5.69291374826433,-4.86935449914238,
5.96847486209515));
#15420=CARTESIAN_POINT('Ctrl Pts',(-5.37211663285,-4.66750507041932,6.02002466665042));
#15421=CARTESIAN_POINT('Ctrl Pts',(-5.16891943289149,-4.39259029914511,
6.06654729043601));
#15422=CARTESIAN_POINT('Ctrl Pts',(-5.08012035782711,-4.06130362216233,
6.11319817659068));
#15423=CARTESIAN_POINT('Ctrl Pts',(-5.118529628433,-3.71945211312213,6.1600007209651));
#15424=CARTESIAN_POINT('Ctrl Pts',(-5.27972004240338,-3.41422893411933,
6.20696368569299));
#15425=CARTESIAN_POINT('Ctrl Pts',(-5.54230107336362,-3.18804339540855,
6.25410140038552));
#15426=CARTESIAN_POINT('Ctrl Pts',(-5.87047888260951,-3.07324172255546,
6.30142586543012));
#15427=CARTESIAN_POINT('Ctrl Pts',(-6.27796878089394,-3.08777452389964,
6.3568679207874));
#15428=CARTESIAN_POINT('Ctrl Pts',(-6.69691616492966,-3.31851514648166,
6.42058411199161));
#15429=CARTESIAN_POINT('Ctrl Pts',(-6.95995510674012,-3.79348275334223,
6.4927626682328));
#15430=CARTESIAN_POINT('Ctrl Pts',(-6.93474143742393,-4.24754819527297,
6.55336750542438));
#15431=CARTESIAN_POINT('Ctrl Pts',(-6.77094422938177,-4.56384857799987,
6.60213386431775));
#15432=CARTESIAN_POINT('Ctrl Pts',(-6.56680914225599,-4.77947610755828,
6.6429345197011));
#15433=CARTESIAN_POINT('Ctrl Pts',(-6.16731733865748,-4.99313041589805,
6.70442493094763));
#15434=CARTESIAN_POINT('Ctrl Pts',(-5.59427289252952,-4.95110526236717,
6.7788227895025));
#15435=CARTESIAN_POINT('Ctrl Pts',(-5.12557736184267,-4.5316246663191,6.86231296849033));
#15436=CARTESIAN_POINT('Ctrl Pts',(-4.9673444927583,-3.98552765323417,6.93810379755276));
#15437=CARTESIAN_POINT('Ctrl Pts',(-5.12600956760141,-3.43315316105931,
7.01455793974746));
#15438=CARTESIAN_POINT('Ctrl Pts',(-5.5573775358164,-3.04671481003938,7.09167935720874));
#15439=CARTESIAN_POINT('Ctrl Pts',(-6.13344795559226,-2.94807981291136,
7.16947389713427));
#15440=CARTESIAN_POINT('Ctrl Pts',(-6.67832238690478,-3.17303200251925,
7.24794018550211));
#15441=CARTESIAN_POINT('Ctrl Pts',(-7.02275755554972,-3.65745608532185,
7.32707217829837));
#15442=CARTESIAN_POINT('Ctrl Pts',(-7.05735272280787,-4.25586588177759,
7.40686459608773));
#15443=CARTESIAN_POINT('Ctrl Pts',(-6.76547691196073,-4.78509631171363,
7.48730845620322));
#15444=CARTESIAN_POINT('Ctrl Pts',(-6.2328288010233,-5.08025350877579,7.56837885030285));
#15445=CARTESIAN_POINT('Ctrl Pts',(-5.62013899574997,-5.04649817639357,
7.65005990391116));
#15446=CARTESIAN_POINT('Ctrl Pts',(-5.11580807772359,-4.68938066411544,
7.73232656442466));
#15447=CARTESIAN_POINT('Ctrl Pts',(-4.87715382894508,-4.11483016176644,
7.81515220419497));
#15448=CARTESIAN_POINT('Ctrl Pts',(-4.98155491462679,-3.49739611646809,
7.89850731279159));
#15449=CARTESIAN_POINT('Ctrl Pts',(-5.40077901066439,-3.02758330352059,
7.9823562570568));
#15450=CARTESIAN_POINT('Ctrl Pts',(-6.00943808507216,-2.85154636954707,
8.06666859923912));
#15451=CARTESIAN_POINT('Ctrl Pts',(-6.51885903425478,-2.99816547885978,
8.1372658921751));
#15452=CARTESIAN_POINT('Ctrl Pts',(-6.83430571931979,-3.26544902128311,
8.19393687266448));
#15453=CARTESIAN_POINT('Ctrl Pts',(-7.05200749163975,-3.59028903861244,
8.24756779276489));
#15454=CARTESIAN_POINT('Ctrl Pts',(-7.14819755856945,-4.06384168275982,
8.31243236873047));
#15455=CARTESIAN_POINT('Ctrl Pts',(-6.98081900179575,-4.60598695891977,
8.38858547422415));
#15456=CARTESIAN_POINT('Ctrl Pts',(-6.60788861986765,-4.97019026806658,
8.458578331888));
#15457=CARTESIAN_POINT('Ctrl Pts',(-6.16543359160979,-5.12466006881932,
8.52232968915992));
#15458=CARTESIAN_POINT('Ctrl Pts',(-5.74359928719466,-5.10906351708155,
8.57978479808564));
#15459=CARTESIAN_POINT('Ctrl Pts',(-5.35619714417686,-4.93996484898772,
8.63729543753528));
#15460=CARTESIAN_POINT('Ctrl Pts',(-5.05707781940967,-4.64089287126633,
8.69485958085149));
#15461=CARTESIAN_POINT('Ctrl Pts',(-4.8877873605468,-4.25294305694932,8.7524561265159));
#15462=CARTESIAN_POINT('Ctrl Pts',(-4.87196688005146,-3.8298677000771,8.81006949812648));
#15463=CARTESIAN_POINT('Ctrl Pts',(-5.01177613480597,-3.43021110565367,
8.86768635580782));
#15464=CARTESIAN_POINT('Ctrl Pts',(-5.28787582930203,-3.10936002434098,
8.92528196146821));
#15465=CARTESIAN_POINT('Ctrl Pts',(-5.6619879756221,-2.91181444586473,8.98285200706347));
#15466=CARTESIAN_POINT('Ctrl Pts',(-6.08207592029199,-2.86437706798175,
9.04037821761112));
#15467=CARTESIAN_POINT('Ctrl Pts',(-6.4899603572735,-2.97385511423952,9.09784598588914));
#15468=CARTESIAN_POINT('Ctrl Pts',(-6.82936497495859,-3.22425165825059,
9.15523814001513));
#15469=CARTESIAN_POINT('Ctrl Pts',(-7.053352906295,-3.58086467861269,9.21254084633562));
#15470=CARTESIAN_POINT('Ctrl Pts',(-7.1313961994424,-3.99398472975135,9.26974226638222));
#15471=CARTESIAN_POINT('Ctrl Pts',(-7.0532945194083,-4.40605187892761,9.32682226439619));
#15472=CARTESIAN_POINT('Ctrl Pts',(-6.80592167656756,-4.800012570465,9.39010214047278));
#15473=CARTESIAN_POINT('Ctrl Pts',(-6.37170927836265,-5.08039142951602,
9.4594993944269));
#15474=CARTESIAN_POINT('Ctrl Pts',(-5.81130091232871,-5.12219506735395,
9.53491939194941));
#15475=CARTESIAN_POINT('Ctrl Pts',(-5.28006160362083,-4.88227948380037,
9.61315239896851));
#15476=CARTESIAN_POINT('Ctrl Pts',(-4.92834155153614,-4.38622356770561,
9.69411365299844));
#15477=CARTESIAN_POINT('Ctrl Pts',(-4.89371133000185,-3.75906326920876,
9.77771093250303));
#15478=CARTESIAN_POINT('Ctrl Pts',(-5.19608243373045,-3.21309740789018,
9.86079489873814));
#15479=CARTESIAN_POINT('Ctrl Pts',(-5.73908153611128,-2.91364502826735,
9.94333398508595));
#15480=CARTESIAN_POINT('Ctrl Pts',(-6.35384329508302,-2.94879350552204,
10.0252993757984));
#15481=CARTESIAN_POINT('Ctrl Pts',(-6.85201080049535,-3.30303898937477,
10.1066658330264));
#15482=CARTESIAN_POINT('Ctrl Pts',(-7.08354371570412,-3.8637384379288,10.187411539775));
#15483=CARTESIAN_POINT('Ctrl Pts',(-6.98206687823625,-4.45694888176359,
10.2675183757904));
#15484=CARTESIAN_POINT('Ctrl Pts',(-6.58379226485485,-4.90158283744291,
10.3469719800326));
#15485=CARTESIAN_POINT('Ctrl Pts',(-6.01478871597461,-5.06478222276206,
10.425761837779));
#15486=CARTESIAN_POINT('Ctrl Pts',(-5.4510073752914,-4.90162602393077,10.5038813791205));
#15487=CARTESIAN_POINT('Ctrl Pts',(-5.06381325555816,-4.46729226158387,
10.581327909048));
#15488=CARTESIAN_POINT('Ctrl Pts',(-4.96788652492998,-3.89849834310758,
10.6581028737864));
#15489=CARTESIAN_POINT('Ctrl Pts',(-5.18737077761513,-3.37046753371988,
10.7342112682679));
#15490=CARTESIAN_POINT('Ctrl Pts',(-5.65010527122599,-3.04297938717396,
10.809662885546));
#15491=CARTESIAN_POINT('Ctrl Pts',(-6.21136781157978,-3.01214055539693,
10.88446936741));
#15492=CARTESIAN_POINT('Ctrl Pts',(-6.69883486154469,-3.28231382194347,
10.9586505197816));
#15493=CARTESIAN_POINT('Ctrl Pts',(-6.96586193433289,-3.7664841398465,11.032219855093));
#15494=CARTESIAN_POINT('Ctrl Pts',(-6.93424119916699,-4.31399510918003,
11.1052163057123));
#15495=CARTESIAN_POINT('Ctrl Pts',(-6.61896949124829,-4.75764538304451,
11.1776579397094));
#15496=CARTESIAN_POINT('Ctrl Pts',(-6.11951941708001,-4.96387158643751,
11.2495798113469));
#15497=CARTESIAN_POINT('Ctrl Pts',(-5.59058419165622,-4.87376112739787,
11.3209980698462));
#15498=CARTESIAN_POINT('Ctrl Pts',(-5.19326858782592,-4.51762113802504,
11.3919960114712));
#15499=CARTESIAN_POINT('Ctrl Pts',(-5.09580224443524,-4.17887730357393,
11.4389949666357));
#15500=CARTESIAN_POINT('Ctrl Pts',(-5.0957793236035,-4.00861533013479,11.462499928691));
#15501=CARTESIAN_POINT('Ctrl Pts',(-4.91064566239329,-3.99023206485658,
2.62933152433034));
#15502=CARTESIAN_POINT('Ctrl Pts',(-4.91067312952917,-3.78619909336401,
2.6574986314607));
#15503=CARTESIAN_POINT('Ctrl Pts',(-5.02774343284091,-3.37929348062033,
2.71396207002513));
#15504=CARTESIAN_POINT('Ctrl Pts',(-5.50406153736764,-2.95270955038751,
2.79904101242933));
#15505=CARTESIAN_POINT('Ctrl Pts',(-6.13658014707958,-2.84513696154089,
2.88444997261576));
#15506=CARTESIAN_POINT('Ctrl Pts',(-6.73146552788189,-3.09119886279762,
2.97014767722273));
#15507=CARTESIAN_POINT('Ctrl Pts',(-7.10528990058372,-3.61770798806037,
3.05608468313627));
#15508=CARTESIAN_POINT('Ctrl Pts',(-7.14159326599711,-4.26367257300153,
3.14221376787915));
#15509=CARTESIAN_POINT('Ctrl Pts',(-6.82847203577308,-4.83116825369024,
3.22848316885409));
#15510=CARTESIAN_POINT('Ctrl Pts',(-6.26047894253337,-5.14498395627411,
3.31484078206362));
#15511=CARTESIAN_POINT('Ctrl Pts',(-5.61243809982754,-5.10862883176423,
3.40123876915193));
#15512=CARTESIAN_POINT('Ctrl Pts',(-5.08312065999899,-4.73301532006664,
3.48762383998782));
#15513=CARTESIAN_POINT('Ctrl Pts',(-4.83503964180896,-4.13383055473192,
3.57394517138351));
#15514=CARTESIAN_POINT('Ctrl Pts',(-4.94365798236383,-3.4953620072643,3.66015124298089));
#15515=CARTESIAN_POINT('Ctrl Pts',(-5.37453812537608,-3.01351481306622,
3.7461917900401));
#15516=CARTESIAN_POINT('Ctrl Pts',(-5.99415503872227,-2.8352869923604,3.83201719977587));
#15517=CARTESIAN_POINT('Ctrl Pts',(-6.61176789561045,-3.01349565884922,
3.91757953433049));
#15518=CARTESIAN_POINT('Ctrl Pts',(-7.02236019753619,-3.47368176991699,
3.99967428100357));
#15519=CARTESIAN_POINT('Ctrl Pts',(-7.11918698593408,-3.95609727910189,
4.06572145278173));
#15520=CARTESIAN_POINT('Ctrl Pts',(-7.06340476330875,-4.27068165104005,
4.10961546484208));
#15521=CARTESIAN_POINT('Ctrl Pts',(-6.99930031338402,-4.44014487854788,
4.13465662034055));
#15522=CARTESIAN_POINT('Ctrl Pts',(-6.87255985096034,-4.68025839089964,
4.17217691756027));
#15523=CARTESIAN_POINT('Ctrl Pts',(-6.57315958771661,-4.97217030656539,
4.22830532196756));
#15524=CARTESIAN_POINT('Ctrl Pts',(-6.03903268776397,-5.12206247506981,
4.30276796426334));
#15525=CARTESIAN_POINT('Ctrl Pts',(-5.50097125621371,-4.99896308035578,
4.37684131892625));
#15526=CARTESIAN_POINT('Ctrl Pts',(-5.12440241748786,-4.66549566032703,
4.44436512761515));
#15527=CARTESIAN_POINT('Ctrl Pts',(-4.94538675915755,-4.2540197256944,4.50542676119247));
#15528=CARTESIAN_POINT('Ctrl Pts',(-4.930305222757,-3.85224640541355,4.56013153880702));
#15529=CARTESIAN_POINT('Ctrl Pts',(-5.06282577996349,-3.47483689360371,
4.61457310279514));
#15530=CARTESIAN_POINT('Ctrl Pts',(-5.35125009676625,-3.1392746316074,4.67476651041697));
#15531=CARTESIAN_POINT('Ctrl Pts',(-5.79829809966802,-2.93804410501286,
4.74058503688818));
#15532=CARTESIAN_POINT('Ctrl Pts',(-6.32807786867545,-2.97826387006224,
4.81188334316262));
#15533=CARTESIAN_POINT('Ctrl Pts',(-6.67840551830293,-3.20520787794476,
4.86793768919777));
#15534=CARTESIAN_POINT('Ctrl Pts',(-6.8595784600443,-3.44180802446728,4.90902136435057));
#15535=CARTESIAN_POINT('Ctrl Pts',(-6.974492766904,-3.66912329852776,4.94413862211746));
#15536=CARTESIAN_POINT('Ctrl Pts',(-7.0340823464101,-3.98480672906872,4.9878512860272));
#15537=CARTESIAN_POINT('Ctrl Pts',(-6.96250196758772,-4.36134912898132,
5.04001006483621));
#15538=CARTESIAN_POINT('Ctrl Pts',(-6.75962908600506,-4.68404810660973,
5.09187209661467));
#15539=CARTESIAN_POINT('Ctrl Pts',(-6.45462282106343,-4.90873382172561,
5.14343601874352));
#15540=CARTESIAN_POINT('Ctrl Pts',(-6.09052764960782,-5.00629817643789,
5.19470121102102));
#15541=CARTESIAN_POINT('Ctrl Pts',(-5.71867585943879,-4.96385753221553,
5.24566987862147));
#15542=CARTESIAN_POINT('Ctrl Pts',(-5.27869458048482,-4.73250913068639,
5.31323392862732));
#15543=CARTESIAN_POINT('Ctrl Pts',(-4.95510149885895,-4.17152363114175,
5.39697303342324));
#15544=CARTESIAN_POINT('Ctrl Pts',(-5.12826577922076,-3.42039982727572,
5.49631984882234));
#15545=CARTESIAN_POINT('Ctrl Pts',(-5.65279054674189,-3.06549368105792,
5.5782074053157));
#15546=CARTESIAN_POINT('Ctrl Pts',(-6.1304657902261,-3.04944345002014,5.64319497079561));
#15547=CARTESIAN_POINT('Ctrl Pts',(-6.50414037104288,-3.17959458133367,
5.69707394622442));
#15548=CARTESIAN_POINT('Ctrl Pts',(-6.81832653237479,-3.4864294509472,5.75599775305137));
#15549=CARTESIAN_POINT('Ctrl Pts',(-6.95798781236734,-3.94133529255923,
5.81987492310173));
#15550=CARTESIAN_POINT('Ctrl Pts',(-6.86406020442495,-4.40486030892628,
5.88336458908467));
#15551=CARTESIAN_POINT('Ctrl Pts',(-6.56145066300743,-4.76499099454252,
5.94650053783697));
#15552=CARTESIAN_POINT('Ctrl Pts',(-6.12579690342053,-4.93562462938296,
6.00930535589766));
#15553=CARTESIAN_POINT('Ctrl Pts',(-5.70231406382442,-4.88235175336122,
6.06660462669795));
#15554=CARTESIAN_POINT('Ctrl Pts',(-5.37955587569654,-4.67904760710474,
6.11850018003562));
#15555=CARTESIAN_POINT('Ctrl Pts',(-5.17633016181025,-4.40380143225806,
6.16506396148214));
#15556=CARTESIAN_POINT('Ctrl Pts',(-5.08810842094241,-4.07402072845824,
6.21150782441348));
#15557=CARTESIAN_POINT('Ctrl Pts',(-5.12629567820714,-3.73567498665909,
6.25783953958017));
#15558=CARTESIAN_POINT('Ctrl Pts',(-5.28511244198756,-3.43529706348013,
6.30407622395686));
#15559=CARTESIAN_POINT('Ctrl Pts',(-5.54229551854319,-3.21398520007125,
6.35023138483534));
#15560=CARTESIAN_POINT('Ctrl Pts',(-5.8619107236865,-3.10233975226692,6.39632010313442));
#15561=CARTESIAN_POINT('Ctrl Pts',(-6.25663673452835,-3.11661537197105,
6.45003081505834));
#15562=CARTESIAN_POINT('Ctrl Pts',(-6.65960184073881,-3.33909366935506,
6.51135170134586));
#15563=CARTESIAN_POINT('Ctrl Pts',(-6.9103998303242,-3.79306634470867,6.58031178132487));
#15564=CARTESIAN_POINT('Ctrl Pts',(-6.88609075922184,-4.22370084373278,
6.63779351550458));
#15565=CARTESIAN_POINT('Ctrl Pts',(-6.73144911525362,-4.5221338311146,6.6838161310143));
#15566=CARTESIAN_POINT('Ctrl Pts',(-6.5394091300997,-4.72493928671578,6.72219558958497));
#15567=CARTESIAN_POINT('Ctrl Pts',(-6.16486636586928,-4.92501555623377,
6.77982471041186));
#15568=CARTESIAN_POINT('Ctrl Pts',(-5.63103734380132,-4.88518117432037,
6.84913849179702));
#15569=CARTESIAN_POINT('Ctrl Pts',(-5.19737626012191,-4.49646149289223,
6.92644120860721));
#15570=CARTESIAN_POINT('Ctrl Pts',(-5.0518312613499,-3.99310443836122,6.99628668811257));
#15571=CARTESIAN_POINT('Ctrl Pts',(-5.1977151858362,-3.48623546915741,7.06644859462949));
#15572=CARTESIAN_POINT('Ctrl Pts',(-5.59236675555469,-3.13299752231314,
7.13697518250154));
#15573=CARTESIAN_POINT('Ctrl Pts',(-6.11768012047296,-3.04324969507249,
7.2079058054426));
#15574=CARTESIAN_POINT('Ctrl Pts',(-6.61330050675189,-3.24802636853269,
7.27928132209));
#15575=CARTESIAN_POINT('Ctrl Pts',(-6.92601453710887,-3.68801965644784,
7.35114007330658));
#15576=CARTESIAN_POINT('Ctrl Pts',(-6.95734111922486,-4.23086268142858,
7.42351372630332));
#15577=CARTESIAN_POINT('Ctrl Pts',(-6.69270416831019,-4.71067464476414,
7.49643069526812));
#15578=CARTESIAN_POINT('Ctrl Pts',(-6.20975100340118,-4.97833378740792,
7.56992638519204));
#15579=CARTESIAN_POINT('Ctrl Pts',(-5.65383497595805,-4.94778246347922,
7.64402199805137));
#15580=CARTESIAN_POINT('Ctrl Pts',(-5.19560892172118,-4.62346526629037,
7.71873991750681));
#15581=CARTESIAN_POINT('Ctrl Pts',(-4.97826933155121,-4.10067068964125,
7.79409718811368));
#15582=CARTESIAN_POINT('Ctrl Pts',(-5.0732790960684,-3.53747137568016,7.87010685457802));
#15583=CARTESIAN_POINT('Ctrl Pts',(-5.45652751621272,-3.10760420604816,
7.94678031881255));
#15584=CARTESIAN_POINT('Ctrl Pts',(-6.01492249584954,-2.94579389365945,
8.02411893674303));
#15585=CARTESIAN_POINT('Ctrl Pts',(-6.48419486025271,-3.08058022325691,
8.08913615817866));
#15586=CARTESIAN_POINT('Ctrl Pts',(-6.77567109544999,-3.32746414120783,
8.14148107252939));
#15587=CARTESIAN_POINT('Ctrl Pts',(-6.97726832362751,-3.62817763584748,
8.19113027512342));
#15588=CARTESIAN_POINT('Ctrl Pts',(-7.06683150986179,-4.06785942369035,
8.25133905297887));
#15589=CARTESIAN_POINT('Ctrl Pts',(-6.91099271737997,-4.57359787784397,
8.32235695721035));
#15590=CARTESIAN_POINT('Ctrl Pts',(-6.56180322265575,-4.91501872365941,
8.38791913097088));
#15591=CARTESIAN_POINT('Ctrl Pts',(-6.1455889673863,-5.06048615843406,8.44788148951164));
#15592=CARTESIAN_POINT('Ctrl Pts',(-5.74726405458259,-5.045901194332,8.5021199776848));
#15593=CARTESIAN_POINT('Ctrl Pts',(-5.37997014596406,-4.88573433422684,
8.55663032383165));
#15594=CARTESIAN_POINT('Ctrl Pts',(-5.09521606139379,-4.60124328031376,
8.61139619541384));
#15595=CARTESIAN_POINT('Ctrl Pts',(-4.93332552837962,-4.23064059662876,
8.66641388088589));
#15596=CARTESIAN_POINT('Ctrl Pts',(-4.9179903715202,-3.82475321029841,8.72167508913329));
#15597=CARTESIAN_POINT('Ctrl Pts',(-5.05253490297233,-3.43967511432446,
8.777169282374));
#15598=CARTESIAN_POINT('Ctrl Pts',(-5.31955851270096,-3.12911022044219,
8.8328932111667));
#15599=CARTESIAN_POINT('Ctrl Pts',(-5.68303528443618,-2.93700186151765,
8.88882890536203));
#15600=CARTESIAN_POINT('Ctrl Pts',(-6.09302465655479,-2.89052402217789,
8.94496765237401));
#15601=CARTESIAN_POINT('Ctrl Pts',(-6.49294269468231,-2.99769732695354,
9.00129753538956));
#15602=CARTESIAN_POINT('Ctrl Pts',(-6.82727292776362,-3.24413114332201,
9.05780821017147));
#15603=CARTESIAN_POINT('Ctrl Pts',(-7.04898730088169,-3.59680786031477,
9.11448652506239));
#15604=CARTESIAN_POINT('Ctrl Pts',(-7.12670330693309,-4.00728190088154,
9.17131792719747));
#15605=CARTESIAN_POINT('Ctrl Pts',(-7.04890710360552,-4.41865064133336,
9.22829293049541));
#15606=CARTESIAN_POINT('Ctrl Pts',(-6.80102480792446,-4.81378239727149,
9.29173772436838));
#15607=CARTESIAN_POINT('Ctrl Pts',(-6.36351538644652,-5.09674069553992,
9.36169115447804));
#15608=CARTESIAN_POINT('Ctrl Pts',(-5.7952165870531,-5.1395532745806,9.43816998078719));
#15609=CARTESIAN_POINT('Ctrl Pts',(-5.25307378945426,-4.89518090505499,
9.51797249895571));
#15610=CARTESIAN_POINT('Ctrl Pts',(-4.89153837004136,-4.38624542537144,
9.60108046017307));
#15611=CARTESIAN_POINT('Ctrl Pts',(-4.85517495180513,-3.73819432300457,
9.68745784720193));
#15612=CARTESIAN_POINT('Ctrl Pts',(-5.16914448740319,-3.17012933555682,
9.77385698474107));
#15613=CARTESIAN_POINT('Ctrl Pts',(-5.73710541159327,-2.85628563202139,
9.86022602760031));
#15614=CARTESIAN_POINT('Ctrl Pts',(-6.38433613751579,-2.89276199039655,
9.94651355241989));
#15615=CARTESIAN_POINT('Ctrl Pts',(-6.91212050930184,-3.26744932078839,
10.0326685712732));
#15616=CARTESIAN_POINT('Ctrl Pts',(-7.15908057305555,-3.86425638646486,
10.1186409109809));
#15617=CARTESIAN_POINT('Ctrl Pts',(-7.05091161244937,-4.49924587495838,
10.2043814658325));
#15618=CARTESIAN_POINT('Ctrl Pts',(-6.62285185241079,-4.97775602995875,
10.2898425301769));
#15619=CARTESIAN_POINT('Ctrl Pts',(-6.00816341099947,-5.15445618405033,
10.3749780585446));
#15620=CARTESIAN_POINT('Ctrl Pts',(-5.39636763024784,-4.97776483774591,
10.4597439223075));
#15621=CARTESIAN_POINT('Ctrl Pts',(-4.97444985106601,-4.50494216067592,
10.5440982117258));
#15622=CARTESIAN_POINT('Ctrl Pts',(-4.86936608454769,-3.88345546663721,
10.62800140343));
#15623=CARTESIAN_POINT('Ctrl Pts',(-5.10968162167462,-3.30472800962943,
10.7114168360999));
#15624=CARTESIAN_POINT('Ctrl Pts',(-5.61787204048362,-2.94485337288711,
10.7943103120336));
#15625=CARTESIAN_POINT('Ctrl Pts',(-6.23553216372117,-2.91079260460954,
10.8766517425954));
#15626=CARTESIAN_POINT('Ctrl Pts',(-6.77273785370402,-3.20844608120544,
10.9584121473814));
#15627=CARTESIAN_POINT('Ctrl Pts',(-7.06723015563896,-3.74240199207279,
11.0395709595654));
#15628=CARTESIAN_POINT('Ctrl Pts',(-7.03232554389622,-4.34631413758613,
11.1201002984029));
#15629=CARTESIAN_POINT('Ctrl Pts',(-6.6846440480935,-4.83541725513737,11.1999834703407));
#15630=CARTESIAN_POINT('Ctrl Pts',(-6.13443860678649,-5.06246468337482,
11.2792177855247));
#15631=CARTESIAN_POINT('Ctrl Pts',(-5.55273853859017,-4.96317392286291,
11.3577768015645));
#15632=CARTESIAN_POINT('Ctrl Pts',(-5.11687440986545,-4.57225551739733,
11.4356905379074));
#15633=CARTESIAN_POINT('Ctrl Pts',(-5.01030571579522,-4.20147270550581,
11.4871432816273));
#15634=CARTESIAN_POINT('Ctrl Pts',(-5.0102806896419,-4.01557184907574,11.5128072187248));
#15635=CARTESIAN_POINT('Ctrl Pts',(-4.97008191124373,-3.98632049867421,
2.60093950625047));
#15636=CARTESIAN_POINT('Ctrl Pts',(-4.97010792325046,-3.79309660191043,
2.62761440178562));
#15637=CARTESIAN_POINT('Ctrl Pts',(-5.08090684239098,-3.40768944058894,
2.68109048286901));
#15638=CARTESIAN_POINT('Ctrl Pts',(-5.53323464929853,-3.00219742821615,
2.76192326014508));
#15639=CARTESIAN_POINT('Ctrl Pts',(-6.13583253713359,-2.89947156896757,
2.84329266550979));
#15640=CARTESIAN_POINT('Ctrl Pts',(-6.70452266565683,-3.13436261802716,
2.92520197170544));
#15641=CARTESIAN_POINT('Ctrl Pts',(-7.06328708852698,-3.63910731072172,
3.00761448887057));
#15642=CARTESIAN_POINT('Ctrl Pts',(-7.09856063711344,-4.26079276792185,
3.09050857590128));
#15643=CARTESIAN_POINT('Ctrl Pts',(-6.79637837460094,-4.80919935005163,
3.17384771454092));
#15644=CARTESIAN_POINT('Ctrl Pts',(-6.24569012974855,-5.11388530829306,
3.25759626910264));
#15645=CARTESIAN_POINT('Ctrl Pts',(-5.61459646028545,-5.07886298559536,
3.34172561849207));
#15646=CARTESIAN_POINT('Ctrl Pts',(-5.09674658023812,-4.71186793716836,
3.4261938545368));
#15647=CARTESIAN_POINT('Ctrl Pts',(-4.85272822511499,-4.1235468329122,3.51096209906644));
#15648=CARTESIAN_POINT('Ctrl Pts',(-4.95946885344308,-3.49366428571328,
3.59598755345742));
#15649=CARTESIAN_POINT('Ctrl Pts',(-5.3860925399307,-3.01594593450921,3.6812267005334));
#15650=CARTESIAN_POINT('Ctrl Pts',(-6.00269019835541,-2.83814374866598,
3.76663475578024));
#15651=CARTESIAN_POINT('Ctrl Pts',(-6.62031834420698,-3.01590617483508,
3.8521649675602));
#15652=CARTESIAN_POINT('Ctrl Pts',(-7.03301623099344,-3.4778365045598,3.93460141464829));
#15653=CARTESIAN_POINT('Ctrl Pts',(-7.13093805843655,-3.96439424471186,
4.00120453997466));
#15654=CARTESIAN_POINT('Ctrl Pts',(-7.07454128905103,-4.28269736823964,
4.04560964054819));
#15655=CARTESIAN_POINT('Ctrl Pts',(-7.00958861255911,-4.45442131099228,
4.07098282756962));
#15656=CARTESIAN_POINT('Ctrl Pts',(-6.88104498689409,-4.69797936078498,
4.10903813285862));
#15657=CARTESIAN_POINT('Ctrl Pts',(-6.57682855326753,-4.99492524656468,
4.1660763537331));
#15658=CARTESIAN_POINT('Ctrl Pts',(-6.0316469704085,-5.14822432672608,4.24208367835567));
#15659=CARTESIAN_POINT('Ctrl Pts',(-5.48021578029777,-5.02235110130459,
4.3179748190391));
#15660=CARTESIAN_POINT('Ctrl Pts',(-5.09271529118042,-4.6795516092149,4.38740377644772));
#15661=CARTESIAN_POINT('Ctrl Pts',(-4.90786994693549,-4.25495657649653,
4.45041036428995));
#15662=CARTESIAN_POINT('Ctrl Pts',(-4.89214664286788,-3.83924497527109,
4.50699930620379));
#15663=CARTESIAN_POINT('Ctrl Pts',(-5.02955352183774,-3.44765692035231,
4.56346991950519));
#15664=CARTESIAN_POINT('Ctrl Pts',(-5.32945197831939,-3.09855693967571,
4.62606391022856));
#15665=CARTESIAN_POINT('Ctrl Pts',(-5.79573806357998,-2.88844341511611,
4.69471397223731));
#15666=CARTESIAN_POINT('Ctrl Pts',(-6.35019247867269,-2.93031759176993,
4.76932252526924));
#15667=CARTESIAN_POINT('Ctrl Pts',(-6.71791383824202,-3.16834791049732,
4.82810753382221));
#15668=CARTESIAN_POINT('Ctrl Pts',(-6.90847162726572,-3.41718092381109,
4.87131014132301));
#15669=CARTESIAN_POINT('Ctrl Pts',(-7.02945840397545,-3.65648859532012,
4.90827460291562));
#15670=CARTESIAN_POINT('Ctrl Pts',(-7.09235415647436,-3.98932316476188,
4.95435468147015));
#15671=CARTESIAN_POINT('Ctrl Pts',(-7.01679613358752,-4.38709288630926,
5.00944049543375));
#15672=CARTESIAN_POINT('Ctrl Pts',(-6.80218102266994,-4.72860976063846,
5.06430748189597));
#15673=CARTESIAN_POINT('Ctrl Pts',(-6.47891565083903,-4.96679436777757,
5.11894822582177));
#15674=CARTESIAN_POINT('Ctrl Pts',(-6.09242502205773,-5.07042049311667,
5.17335860716689));
#15675=CARTESIAN_POINT('Ctrl Pts',(-5.69712814211187,-5.02533685252607,
5.22752916796423));
#15676=CARTESIAN_POINT('Ctrl Pts',(-5.22881038622497,-4.77916247689946,
5.29943193022554));
#15677=CARTESIAN_POINT('Ctrl Pts',(-4.8836815835944,-4.18127755734618,5.38866309511102));
#15678=CARTESIAN_POINT('Ctrl Pts',(-5.06839094832227,-3.37929873201119,
5.49470580468442));
#15679=CARTESIAN_POINT('Ctrl Pts',(-5.62883774530645,-3.00003776994351,
5.58217611826977));
#15680=CARTESIAN_POINT('Ctrl Pts',(-6.13932551294608,-2.98290693407233,
5.65161646350273));
#15681=CARTESIAN_POINT('Ctrl Pts',(-6.53861788941739,-3.12198633810778,
5.70918134513565));
#15682=CARTESIAN_POINT('Ctrl Pts',(-6.8742032976184,-3.4497749510831,5.77211341790662));
#15683=CARTESIAN_POINT('Ctrl Pts',(-7.02320804724903,-3.93535711597183,
5.84028217731445));
#15684=CARTESIAN_POINT('Ctrl Pts',(-6.92297139477486,-4.42960801271712,
5.90797662474841));
#15685=CARTESIAN_POINT('Ctrl Pts',(-6.60065686050615,-4.81301742724568,
5.97519783526073));
#15686=CARTESIAN_POINT('Ctrl Pts',(-6.13749803630879,-4.99428816457585,
6.04195679074869));
#15687=CARTESIAN_POINT('Ctrl Pts',(-5.68826175552714,-4.9376390353816,6.1027374472312));
#15688=CARTESIAN_POINT('Ctrl Pts',(-5.34662282232589,-4.7223338410458,6.15767181180174));
#15689=CARTESIAN_POINT('Ctrl Pts',(-5.13194361739086,-4.43145703525003,
6.20687182350689));
#15690=CARTESIAN_POINT('Ctrl Pts',(-5.03901270494996,-4.08371896980411,
6.25583828963203));
#15691=CARTESIAN_POINT('Ctrl Pts',(-5.07927303344496,-3.72779634187791,
6.30457776363547));
#15692=CARTESIAN_POINT('Ctrl Pts',(-5.24602249926503,-3.41261874140077,
6.35309845686694));
#15693=CARTESIAN_POINT('Ctrl Pts',(-5.5152804095074,-3.1810516668998,6.40140936712654));
#15694=CARTESIAN_POINT('Ctrl Pts',(-5.84893154516085,-3.06460741415626,
6.44951841989009));
#15695=CARTESIAN_POINT('Ctrl Pts',(-6.25977592394247,-3.07960237391109,
6.50542489105098));
#15696=CARTESIAN_POINT('Ctrl Pts',(-6.67746012847371,-3.31055664624366,
6.56900781660853));
#15697=CARTESIAN_POINT('Ctrl Pts',(-6.93590942148792,-3.77925425753501,
6.64018638784732));
#15698=CARTESIAN_POINT('Ctrl Pts',(-6.91063838592921,-4.22138495835218,
6.69920846194775));
#15699=CARTESIAN_POINT('Ctrl Pts',(-6.75240356125144,-4.52656025392589,
6.74628493506968));
#15700=CARTESIAN_POINT('Ctrl Pts',(-6.55648751063966,-4.73340807548516,
6.78543807765367));
#15701=CARTESIAN_POINT('Ctrl Pts',(-6.17549659731643,-4.93670212163746,
6.84404533283986));
#15702=CARTESIAN_POINT('Ctrl Pts',(-5.63568864954653,-4.89574010065246,
6.91414579643729));
#15703=CARTESIAN_POINT('Ctrl Pts',(-5.20029791031333,-4.50472944721903,
6.99184586086499));
#15704=CARTESIAN_POINT('Ctrl Pts',(-5.05524611097297,-4.0016492232368,7.06165065576445));
#15705=CARTESIAN_POINT('Ctrl Pts',(-5.20062622496947,-3.49805247371584,
7.13139550084469));
#15706=CARTESIAN_POINT('Ctrl Pts',(-5.59091658743601,-3.14926506675406,
7.20110582590366));
#15707=CARTESIAN_POINT('Ctrl Pts',(-6.10736329715364,-3.06142476350215,
7.27084568737173));
#15708=CARTESIAN_POINT('Ctrl Pts',(-6.59186085954437,-3.26202265988594,
7.34065571252636));
#15709=CARTESIAN_POINT('Ctrl Pts',(-6.89581340654691,-3.69030143654108,
7.41058101647453));
#15710=CARTESIAN_POINT('Ctrl Pts',(-6.92579082783416,-4.21593899400802,
7.48067473906963));
#15711=CARTESIAN_POINT('Ctrl Pts',(-6.67042532145853,-4.67827675202706,
7.55099101068251));
#15712=CARTESIAN_POINT('Ctrl Pts',(-6.20676421941765,-4.93489381099811,
7.621551806708));
#15713=CARTESIAN_POINT('Ctrl Pts',(-5.67535748365785,-4.90541034209074,
7.69240985629438));
#15714=CARTESIAN_POINT('Ctrl Pts',(-5.23906347903042,-4.5962956089863,7.76360171950934));
#15715=CARTESIAN_POINT('Ctrl Pts',(-5.03295148115901,-4.0998893028727,7.8351675530826));
#15716=CARTESIAN_POINT('Ctrl Pts',(-5.12310040907612,-3.56680199598165,
7.90714445094969));
#15717=CARTESIAN_POINT('Ctrl Pts',(-5.48510203815549,-3.16103430736412,
7.97956372049517));
#15718=CARTESIAN_POINT('Ctrl Pts',(-6.01128256578978,-3.00871765656471,
8.0524644644889));
#15719=CARTESIAN_POINT('Ctrl Pts',(-6.45259276873704,-3.13557676936373,
8.11361809715538));
#15720=CARTESIAN_POINT('Ctrl Pts',(-6.72644062352849,-3.3675500016554,8.16281094434981));
#15721=CARTESIAN_POINT('Ctrl Pts',(-6.91573050923383,-3.64992945061337,
8.20943672508966));
#15722=CARTESIAN_POINT('Ctrl Pts',(-6.9997439667954,-4.06259387267818,8.26596983287103));
#15723=CARTESIAN_POINT('Ctrl Pts',(-6.85357445098635,-4.5369172654714,8.33258593322727));
#15724=CARTESIAN_POINT('Ctrl Pts',(-6.52613326631928,-4.85706075770687,
8.39407600868389));
#15725=CARTESIAN_POINT('Ctrl Pts',(-6.13582429272564,-4.99349511886135,
8.4503205266024));
#15726=CARTESIAN_POINT('Ctrl Pts',(-5.76219860171794,-4.97982687279222,
8.50120815835136));
#15727=CARTESIAN_POINT('Ctrl Pts',(-5.41756394793594,-4.82956789187536,
8.55235995770513));
#15728=CARTESIAN_POINT('Ctrl Pts',(-5.15020706355995,-4.56249213532047,
8.60378685083323));
#15729=CARTESIAN_POINT('Ctrl Pts',(-4.9980806986773,-4.21432615798783,8.65548587532449));
#15730=CARTESIAN_POINT('Ctrl Pts',(-4.98362078138167,-3.83267457667929,
8.70745682142475));
#15731=CARTESIAN_POINT('Ctrl Pts',(-5.11021173610357,-3.47020564084564,
8.75970064885389));
#15732=CARTESIAN_POINT('Ctrl Pts',(-5.36178391702095,-3.17754370452478,
8.81221057010265));
#15733=CARTESIAN_POINT('Ctrl Pts',(-5.70469395829501,-2.99623679778711,
8.86499141460679));
#15734=CARTESIAN_POINT('Ctrl Pts',(-6.09205813677498,-2.95226910744711,
8.91803745092096));
#15735=CARTESIAN_POINT('Ctrl Pts',(-6.47051636999889,-3.05361664512734,
8.9713474017782));
#15736=CARTESIAN_POINT('Ctrl Pts',(-6.78745601078875,-3.2871476120119,9.02491490657847));
#15737=CARTESIAN_POINT('Ctrl Pts',(-6.99804991983352,-3.6219905623486,9.07873698274717));
#15738=CARTESIAN_POINT('Ctrl Pts',(-7.07207026168852,-4.01248712098153,
9.13280775366998));
#15739=CARTESIAN_POINT('Ctrl Pts',(-6.99798838023044,-4.40464589014135,
9.18712123173382));
#15740=CARTESIAN_POINT('Ctrl Pts',(-6.76128106236067,-4.78216208475497,
9.24773154241494));
#15741=CARTESIAN_POINT('Ctrl Pts',(-6.34236359791613,-5.05332459558266,
9.31472994340359));
#15742=CARTESIAN_POINT('Ctrl Pts',(-5.79640293018885,-5.09468728035619,
9.38820557688175));
#15743=CARTESIAN_POINT('Ctrl Pts',(-5.27374807194744,-4.85938295343188,
9.46512285630086));
#15744=CARTESIAN_POINT('Ctrl Pts',(-4.92374139291998,-4.36727160302241,
9.54551374515351));
#15745=CARTESIAN_POINT('Ctrl Pts',(-4.88804833882704,-3.73790823726897,
9.62939856567637));
#15746=CARTESIAN_POINT('Ctrl Pts',(-5.19389456911797,-3.18374459916885,
9.7136487215973));
#15747=CARTESIAN_POINT('Ctrl Pts',(-5.7499262029823,-2.87603897724937,9.79822511636517));
#15748=CARTESIAN_POINT('Ctrl Pts',(-6.38655698857843,-2.91151088221277,
9.88308689374091));
#15749=CARTESIAN_POINT('Ctrl Pts',(-6.90821328840495,-3.28134043117039,
9.96819148980261));
#15750=CARTESIAN_POINT('Ctrl Pts',(-7.15367511216456,-3.87342998538574,
10.0534949279284));
#15751=CARTESIAN_POINT('Ctrl Pts',(-7.04626285151201,-4.50649326011972,
10.1389520349226));
#15752=CARTESIAN_POINT('Ctrl Pts',(-6.61792394699237,-4.98595040081837,
10.2245167629568));
#15753=CARTESIAN_POINT('Ctrl Pts',(-5.99969540032943,-5.16410689978942,
10.3101423900334));
#15754=CARTESIAN_POINT('Ctrl Pts',(-5.38135114053038,-4.98595903034396,
10.3957818820093));
#15755=CARTESIAN_POINT('Ctrl Pts',(-4.95276973155278,-4.50628650839756,
10.4813879625181));
#15756=CARTESIAN_POINT('Ctrl Pts',(-4.84522951556671,-3.87269630342893,
10.5669138370986));
#15757=CARTESIAN_POINT('Ctrl Pts',(-5.09095827763592,-3.27990007927789,
10.6523125070039));
#15758=CARTESIAN_POINT('Ctrl Pts',(-5.61337048591891,-2.90947965858988,
10.7375390455524));
#15759=CARTESIAN_POINT('Ctrl Pts',(-6.2512116652945,-2.8739197839433,10.8225463831617));
#15760=CARTESIAN_POINT('Ctrl Pts',(-6.80839117558467,-3.18222380258799,
10.9072955143056));
#15761=CARTESIAN_POINT('Ctrl Pts',(-7.11523129697893,-3.73778673767215,
10.9917334063949));
#15762=CARTESIAN_POINT('Ctrl Pts',(-7.07909456599979,-4.36871911225707,
11.0758426906577));
#15763=CARTESIAN_POINT('Ctrl Pts',(-6.71487307508494,-4.88164185779045,
11.1595743427241));
#15764=CARTESIAN_POINT('Ctrl Pts',(-6.13633158216785,-5.12070793186404,
11.2428882077646));
#15765=CARTESIAN_POINT('Ctrl Pts',(-5.52270076886875,-5.01618598996208,
11.325745296715));
#15766=CARTESIAN_POINT('Ctrl Pts',(-5.06153326945952,-4.60290245400468,
11.4081370879796));
#15767=CARTESIAN_POINT('Ctrl Pts',(-4.94849818871498,-4.20962129150326,
11.4626969504328));
#15768=CARTESIAN_POINT('Ctrl Pts',(-4.94847164137574,-4.01242066547175,
11.4899208404097));
#15769=CARTESIAN_POINT('Ctrl Pts',(-5.0000018410068,-3.98632452652701,2.60093950625047));
#15770=CARTESIAN_POINT('Ctrl Pts',(-5.00002711936198,-3.79855038268961,
2.62686205390092));
#15771=CARTESIAN_POINT('Ctrl Pts',(-5.10766548646186,-3.42414266353048,
2.67881373981085));
#15772=CARTESIAN_POINT('Ctrl Pts',(-5.54728618664091,-3.02997941177219,
2.75738438838345));
#15773=CARTESIAN_POINT('Ctrl Pts',(-6.13328094577175,-2.93005881251319,
2.83651316903494));
#15774=CARTESIAN_POINT('Ctrl Pts',(-6.68670283260197,-3.15858336118752,
2.91622304878198));
#15775=CARTESIAN_POINT('Ctrl Pts',(-7.03616187921695,-3.65012597802659,
2.99648821676135));
#15776=CARTESIAN_POINT('Ctrl Pts',(-7.07062949516082,-4.25616589762635,
3.07729930317819));
#15777=CARTESIAN_POINT('Ctrl Pts',(-6.77580863517498,-4.79139923899731,
3.15863489698049));
#15778=CARTESIAN_POINT('Ctrl Pts',(-6.23777999713871,-5.08919902934938,
3.24047455745509));
#15779=CARTESIAN_POINT('Ctrl Pts',(-5.62032344264714,-5.05504677509261,
3.32279321070673));
#15780=CARTESIAN_POINT('Ctrl Pts',(-5.11287137916696,-4.69557478020053,
3.40556356877954));
#15781=CARTESIAN_POINT('Ctrl Pts',(-4.87329914702911,-4.11831903637453,
3.48875540125931));
#15782=CARTESIAN_POINT('Ctrl Pts',(-4.97807346419814,-3.49920456570944,
3.57233609900605));
#15783=CARTESIAN_POINT('Ctrl Pts',(-5.39799493781825,-3.02877333945258,
3.65627071903615));
#15784=CARTESIAN_POINT('Ctrl Pts',(-6.00610273172108,-2.85326324045065,
3.74052224127624));
#15785=CARTESIAN_POINT('Ctrl Pts',(-6.61643757836359,-3.02876545098225,
3.82505176791358));
#15786=CARTESIAN_POINT('Ctrl Pts',(-7.02513160270699,-3.48597574268572,
3.90667922493066));
#15787=CARTESIAN_POINT('Ctrl Pts',(-7.12235641775929,-3.9685483460108,3.97275270898905));
#15788=CARTESIAN_POINT('Ctrl Pts',(-7.06636481269846,-4.28466100128236,
4.01685604551847));
#15789=CARTESIAN_POINT('Ctrl Pts',(-7.00182040328561,-4.45530975229043,
4.04207155819959));
#15790=CARTESIAN_POINT('Ctrl Pts',(-6.87402691871924,-4.69744869614318,
4.07990746733096));
#15791=CARTESIAN_POINT('Ctrl Pts',(-6.57124878899927,-4.99309357202046,
4.1367051149187));
#15792=CARTESIAN_POINT('Ctrl Pts',(-6.02768033690931,-5.14605913758532,
4.2124974864954));
#15793=CARTESIAN_POINT('Ctrl Pts',(-5.47679456345111,-5.0204436702095,4.28832048286543));
#15794=CARTESIAN_POINT('Ctrl Pts',(-5.08889541312948,-4.67743201497751,
4.35782392862843));
#15795=CARTESIAN_POINT('Ctrl Pts',(-4.90355272665998,-4.25185719379132,
4.42098501738742));
#15796=CARTESIAN_POINT('Ctrl Pts',(-4.88772422317122,-3.83457870292561,
4.47779828347438));
#15797=CARTESIAN_POINT('Ctrl Pts',(-5.02577825319216,-3.44096047951616,
4.5345666000236));
#15798=CARTESIAN_POINT('Ctrl Pts',(-5.32758243531257,-3.08955719770179,
4.59757801626674));
#15799=CARTESIAN_POINT('Ctrl Pts',(-5.79757132369034,-2.87764760865861,
4.66678930745632));
#15800=CARTESIAN_POINT('Ctrl Pts',(-6.35748141231083,-2.91980778121556,
4.74213608943437));
#15801=CARTESIAN_POINT('Ctrl Pts',(-6.72958410590507,-3.16055362161142,
4.80163845366161));
#15802=CARTESIAN_POINT('Ctrl Pts',(-6.922583408066,-3.41255717151317,4.8453962925926));
#15803=CARTESIAN_POINT('Ctrl Pts',(-7.04520229026909,-3.65506744231538,
4.88286085267916));
#15804=CARTESIAN_POINT('Ctrl Pts',(-7.10903827020174,-3.9926759490213,4.92960885619655));
#15805=CARTESIAN_POINT('Ctrl Pts',(-7.032354492376,-4.39667067923105,4.98556279568034));
#15806=CARTESIAN_POINT('Ctrl Pts',(-6.81415974257675,-4.74396102273289,
5.04136211338037));
#15807=CARTESIAN_POINT('Ctrl Pts',(-6.48510242262688,-4.98648342248571,
5.09699623581333));
#15808=CARTESIAN_POINT('Ctrl Pts',(-6.09122164110091,-5.09213718968761,
5.15245506498449));
#15809=CARTESIAN_POINT('Ctrl Pts',(-5.6879156360413,-5.04618557814476,5.20772889788153));
#15810=CARTESIAN_POINT('Ctrl Pts',(-5.20960410281967,-4.79482820495352,
5.28116853491036));
#15811=CARTESIAN_POINT('Ctrl Pts',(-4.85635661256684,-4.18339627204868,
5.37246079310469));
#15812=CARTESIAN_POINT('Ctrl Pts',(-5.04534497366866,-3.36152922837358,
5.4811368047244));
#15813=CARTESIAN_POINT('Ctrl Pts',(-5.62045222073828,-2.97210695679973,
5.57092649482181));
#15814=CARTESIAN_POINT('Ctrl Pts',(-6.14491401311764,-2.95446524901901,
5.64227218329944));
#15815=CARTESIAN_POINT('Ctrl Pts',(-6.55538629310792,-3.09741218079302,
5.70145206897501));
#15816=CARTESIAN_POINT('Ctrl Pts',(-6.90061904209687,-3.43455608810828,
5.76619150175189));
#15817=CARTESIAN_POINT('Ctrl Pts',(-7.05403180026006,-3.93434682913999,
5.83636208061574));
#15818=CARTESIAN_POINT('Ctrl Pts',(-6.95084370870626,-4.44331194962687,
5.90607316768221));
#15819=CARTESIAN_POINT('Ctrl Pts',(-6.61884201115902,-4.83828819326241,
5.97532164622816));
#15820=CARTESIAN_POINT('Ctrl Pts',(-6.14163977231472,-5.02507153362565,
6.04410658214742));
#15821=CARTESIAN_POINT('Ctrl Pts',(-5.67874308979945,-4.96670943531882,
6.10673565115305));
#15822=CARTESIAN_POINT('Ctrl Pts',(-5.32673727495899,-4.74487796933182,
6.16333654805419));
#15823=CARTESIAN_POINT('Ctrl Pts',(-5.10557737295403,-4.44521639081723,
6.21402149420468));
#15824=CARTESIAN_POINT('Ctrl Pts',(-5.00986236436416,-4.08706033297606,
6.26445344628883));
#15825=CARTESIAN_POINT('Ctrl Pts',(-5.05132140869747,-3.72058500062059,
6.31463598386295));
#15826=CARTESIAN_POINT('Ctrl Pts',(-5.22295427342147,-3.39619318419661,
6.36457331207659));
#15827=CARTESIAN_POINT('Ctrl Pts',(-5.49996349858563,-3.15797332202467,
6.41427030413784));
#15828=CARTESIAN_POINT('Ctrl Pts',(-5.843023257891,-3.03825996963253,6.46373244033231));
#15829=CARTESIAN_POINT('Ctrl Pts',(-6.2651798733637,-3.05368284090179,6.52117143934356));
#15830=CARTESIAN_POINT('Ctrl Pts',(-6.69395218073661,-3.29085487418832,
6.58644589644131));
#15831=CARTESIAN_POINT('Ctrl Pts',(-6.9588514090406,-3.77142724594311,6.65940509135759));
#15832=CARTESIAN_POINT('Ctrl Pts',(-6.93289301903251,-4.22410112506723,
6.71983222544231));
#15833=CARTESIAN_POINT('Ctrl Pts',(-6.77106481048377,-4.53615877260298,
6.76796591761938));
#15834=CARTESIAN_POINT('Ctrl Pts',(-6.57088599598262,-4.74749645053629,
6.8079662999785));
#15835=CARTESIAN_POINT('Ctrl Pts',(-6.18196007039062,-4.95496402481898,
6.86778079666891));
#15836=CARTESIAN_POINT('Ctrl Pts',(-5.63200940413013,-4.91297894303413,
6.93919834468442));
#15837=CARTESIAN_POINT('Ctrl Pts',(-5.18963313111942,-4.51545599119052,
7.01814869825501));
#15838=CARTESIAN_POINT('Ctrl Pts',(-5.04266994609727,-4.00519996765647,
7.08893288548598));
#15839=CARTESIAN_POINT('Ctrl Pts',(-5.18994160065279,-3.49569082009585,
7.15948665627275));
#15840=CARTESIAN_POINT('Ctrl Pts',(-5.58406477811046,-3.14370617953113,
7.22985222522876));
#15841=CARTESIAN_POINT('Ctrl Pts',(-6.10419876841606,-3.05543002721108,
7.30007283323036));
#15842=CARTESIAN_POINT('Ctrl Pts',(-6.59085610258569,-3.25712241290123,
7.37019262147636));
#15843=CARTESIAN_POINT('Ctrl Pts',(-6.8952969281062,-3.68642062054244,7.44025632508636));
#15844=CARTESIAN_POINT('Ctrl Pts',(-6.92507910037993,-4.2118623997588,7.51030900497373));
#15845=CARTESIAN_POINT('Ctrl Pts',(-6.67029196164112,-4.6727438878236,7.58039577683535));
#15846=CARTESIAN_POINT('Ctrl Pts',(-6.20902606294958,-4.92782413963266,
7.65056157433059));
#15847=CARTESIAN_POINT('Ctrl Pts',(-5.68175068955988,-4.89838259463549,
7.72085085746158));
#15848=CARTESIAN_POINT('Ctrl Pts',(-5.24995696526907,-4.59224234497362,
7.79130734612191));
#15849=CARTESIAN_POINT('Ctrl Pts',(-5.04653976812282,-4.10189023096155,
7.86197377554524));
#15850=CARTESIAN_POINT('Ctrl Pts',(-5.13553771446182,-3.57654536818086,
7.93289164421975));
#15851=CARTESIAN_POINT('Ctrl Pts',(-5.49167958880606,-3.17757206270347,
8.00410097016463));
#15852=CARTESIAN_POINT('Ctrl Pts',(-6.00820878856796,-3.02820291673281,
8.07564000225066));
#15853=CARTESIAN_POINT('Ctrl Pts',(-6.44062187419601,-3.15261370888403,
8.13556092469148));
#15854=CARTESIAN_POINT('Ctrl Pts',(-6.70861130655355,-3.37965195671477,
8.18369776363854));
#15855=CARTESIAN_POINT('Ctrl Pts',(-6.8937105085998,-3.65581236490976,8.22929135600403));
#15856=CARTESIAN_POINT('Ctrl Pts',(-6.97571459288556,-4.05892831151958,
8.28449961702882));
#15857=CARTESIAN_POINT('Ctrl Pts',(-6.83301647708075,-4.52172879570838,
8.34949564023339));
#15858=CARTESIAN_POINT('Ctrl Pts',(-6.51381452164907,-4.83374162454526,
8.40942447333573));
#15859=CARTESIAN_POINT('Ctrl Pts',(-6.13367096105595,-4.96658596055631,
8.46419547642941));
#15860=CARTESIAN_POINT('Ctrl Pts',(-5.77000769054747,-4.95325944490059,
8.51371979160536));
#15861=CARTESIAN_POINT('Ctrl Pts',(-5.43473421944715,-4.80705755452014,
8.56348049202891));
#15862=CARTESIAN_POINT('Ctrl Pts',(-5.17476962038704,-4.5473411130966,8.6134828902317));
#15863=CARTESIAN_POINT('Ctrl Pts',(-5.02691233865341,-4.20890181210803,
8.66373168353468));
#15864=CARTESIAN_POINT('Ctrl Pts',(-5.01287597198371,-3.83802632501149,
8.71423091550292));
#15865=CARTESIAN_POINT('Ctrl Pts',(-5.13588065841094,-3.48587318149708,
8.76498396862734));
#15866=CARTESIAN_POINT('Ctrl Pts',(-5.38027484984219,-3.20156985271231,
8.81599355960519));
#15867=CARTESIAN_POINT('Ctrl Pts',(-5.71337748308179,-3.0254571982762,8.86726173709343));
#15868=CARTESIAN_POINT('Ctrl Pts',(-6.08966550245643,-2.98274869856715,
8.91878984711541));
#15869=CARTESIAN_POINT('Ctrl Pts',(-6.45733798876018,-3.0812109148485,8.97057858675351));
#15870=CARTESIAN_POINT('Ctrl Pts',(-6.76529910592523,-3.30812336168265,
9.02262792849601));
#15871=CARTESIAN_POINT('Ctrl Pts',(-6.96998046112789,-3.63355675694242,
9.07493719450744));
#15872=CARTESIAN_POINT('Ctrl Pts',(-7.04194989283072,-4.01319995364602,
9.12750500078302));
#15873=CARTESIAN_POINT('Ctrl Pts',(-6.96991048459342,-4.39460760383808,
9.18032929219698));
#15874=CARTESIAN_POINT('Ctrl Pts',(-6.73960211403654,-4.76194359718324,
9.23930488555841));
#15875=CARTESIAN_POINT('Ctrl Pts',(-6.33176853957225,-5.02597941464994,
9.30453505646424));
#15876=CARTESIAN_POINT('Ctrl Pts',(-5.79980377218573,-5.06633098935627,
9.37613051632468));
#15877=CARTESIAN_POINT('Ctrl Pts',(-5.29005475531646,-4.836901018808,9.45115010972279));
#15878=CARTESIAN_POINT('Ctrl Pts',(-4.94827191401131,-4.35650564743655,
9.52964181326016));
#15879=CARTESIAN_POINT('Ctrl Pts',(-4.91327405487842,-3.74129847888372,
9.61164803952703));
#15880=CARTESIAN_POINT('Ctrl Pts',(-5.21254904956895,-3.19880095424663,
9.69412425066449));
#15881=CARTESIAN_POINT('Ctrl Pts',(-5.75755518053287,-2.89705290752891,
9.77704206923956));
#15882=CARTESIAN_POINT('Ctrl Pts',(-6.38261532053777,-2.93174547355756,
9.86037047436186));
#15883=CARTESIAN_POINT('Ctrl Pts',(-6.89571246871018,-3.29533246954376,
9.9440760489684));
#15884=CARTESIAN_POINT('Ctrl Pts',(-7.13766462222267,-3.87856431327716,
10.0281231253342));
#15885=CARTESIAN_POINT('Ctrl Pts',(-7.03181307520858,-4.50336859593469,
10.112474009291));
#15886=CARTESIAN_POINT('Ctrl Pts',(-6.60841405754483,-4.9775421382096,10.1970892234063));
#15887=CARTESIAN_POINT('Ctrl Pts',(-5.99601356400164,-5.15419586953956,
10.2819277209876));
#15888=CARTESIAN_POINT('Ctrl Pts',(-5.38220054085499,-4.97753568370925,
10.3669471364924));
#15889=CARTESIAN_POINT('Ctrl Pts',(-4.95580917322647,-4.50058383383181,
10.4521040148979));
#15890=CARTESIAN_POINT('Ctrl Pts',(-4.84845524689304,-3.86918295104257,
10.5373541217208));
#15891=CARTESIAN_POINT('Ctrl Pts',(-5.09367725879538,-3.27712852401529,
10.6226526455382));
#15892=CARTESIAN_POINT('Ctrl Pts',(-5.6163401918585,-2.90630478068196,10.7079544990261));
#15893=CARTESIAN_POINT('Ctrl Pts',(-6.25592072702474,-2.87046899980689,
10.7932145516894));
#15894=CARTESIAN_POINT('Ctrl Pts',(-6.81586294759382,-3.18009679237689,
10.8783879977619));
#15895=CARTESIAN_POINT('Ctrl Pts',(-7.124955642463,-3.73939634942269,10.963430385322));
#15896=CARTESIAN_POINT('Ctrl Pts',(-7.08867264951758,-4.37593520057008,
11.0482983435205));
#15897=CARTESIAN_POINT('Ctrl Pts',(-6.72062823969146,-4.89450906450982,
11.1329488746335));
#15898=CARTESIAN_POINT('Ctrl Pts',(-6.13472454520284,-5.136799701332,11.217341733611));
#15899=CARTESIAN_POINT('Ctrl Pts',(-5.51200536776972,-5.03087324497862,
11.3014349939178));
#15900=CARTESIAN_POINT('Ctrl Pts',(-5.04306930328679,-4.6109089567958,11.3851957518917));
#15901=CARTESIAN_POINT('Ctrl Pts',(-4.92780437314592,-4.2103503377694,11.4407823887583));
#15902=CARTESIAN_POINT('Ctrl Pts',(-4.92777733020741,-4.00946826990451,
11.4685145081939));
#15903=CARTESIAN_POINT('',(-5.0000018410068,-3.98632452652701,2.60093950625047));
#15904=CARTESIAN_POINT('Origin',(-5.,-4.,2.7));
#15905=CARTESIAN_POINT('',(-4.92777733020741,-4.00946826990451,11.4685145081939));
#15906=CARTESIAN_POINT('Ctrl Pts',(-5.0000018410068,-3.98632452652701,2.60093950625047));
#15907=CARTESIAN_POINT('Ctrl Pts',(-5.00002711936198,-3.79855038268961,
2.62686205390092));
#15908=CARTESIAN_POINT('Ctrl Pts',(-5.10766548646186,-3.42414266353048,
2.67881373981085));
#15909=CARTESIAN_POINT('Ctrl Pts',(-5.54728618664091,-3.02997941177219,
2.75738438838345));
#15910=CARTESIAN_POINT('Ctrl Pts',(-6.13328094577175,-2.93005881251319,
2.83651316903494));
#15911=CARTESIAN_POINT('Ctrl Pts',(-6.68670283260197,-3.15858336118752,
2.91622304878198));
#15912=CARTESIAN_POINT('Ctrl Pts',(-7.03616187921695,-3.65012597802659,
2.99648821676135));
#15913=CARTESIAN_POINT('Ctrl Pts',(-7.07062949516082,-4.25616589762635,
3.07729930317819));
#15914=CARTESIAN_POINT('Ctrl Pts',(-6.77580863517498,-4.79139923899731,
3.15863489698049));
#15915=CARTESIAN_POINT('Ctrl Pts',(-6.23777999713871,-5.08919902934938,
3.24047455745509));
#15916=CARTESIAN_POINT('Ctrl Pts',(-5.62032344264714,-5.05504677509261,
3.32279321070673));
#15917=CARTESIAN_POINT('Ctrl Pts',(-5.11287137916696,-4.69557478020053,
3.40556356877954));
#15918=CARTESIAN_POINT('Ctrl Pts',(-4.87329914702911,-4.11831903637453,
3.48875540125931));
#15919=CARTESIAN_POINT('Ctrl Pts',(-4.97807346419814,-3.49920456570944,
3.57233609900605));
#15920=CARTESIAN_POINT('Ctrl Pts',(-5.39799493781825,-3.02877333945258,
3.65627071903615));
#15921=CARTESIAN_POINT('Ctrl Pts',(-6.00610273172108,-2.85326324045065,
3.74052224127624));
#15922=CARTESIAN_POINT('Ctrl Pts',(-6.61643757836359,-3.02876545098225,
3.82505176791358));
#15923=CARTESIAN_POINT('Ctrl Pts',(-7.02513160270699,-3.48597574268572,
3.90667922493066));
#15924=CARTESIAN_POINT('Ctrl Pts',(-7.12235641775929,-3.9685483460108,3.97275270898905));
#15925=CARTESIAN_POINT('Ctrl Pts',(-7.06636481269846,-4.28466100128236,
4.01685604551847));
#15926=CARTESIAN_POINT('Ctrl Pts',(-7.00182040328561,-4.45530975229043,
4.04207155819959));
#15927=CARTESIAN_POINT('Ctrl Pts',(-6.87402691871924,-4.69744869614318,
4.07990746733096));
#15928=CARTESIAN_POINT('Ctrl Pts',(-6.57124878899927,-4.99309357202046,
4.1367051149187));
#15929=CARTESIAN_POINT('Ctrl Pts',(-6.02768033690931,-5.14605913758532,
4.2124974864954));
#15930=CARTESIAN_POINT('Ctrl Pts',(-5.47679456345111,-5.0204436702095,4.28832048286543));
#15931=CARTESIAN_POINT('Ctrl Pts',(-5.08889541312948,-4.67743201497751,
4.35782392862843));
#15932=CARTESIAN_POINT('Ctrl Pts',(-4.90355272665998,-4.25185719379132,
4.42098501738742));
#15933=CARTESIAN_POINT('Ctrl Pts',(-4.88772422317122,-3.83457870292561,
4.47779828347438));
#15934=CARTESIAN_POINT('Ctrl Pts',(-5.02577825319216,-3.44096047951616,
4.5345666000236));
#15935=CARTESIAN_POINT('Ctrl Pts',(-5.32758243531257,-3.08955719770179,
4.59757801626674));
#15936=CARTESIAN_POINT('Ctrl Pts',(-5.79757132369034,-2.87764760865861,
4.66678930745632));
#15937=CARTESIAN_POINT('Ctrl Pts',(-6.35748141231083,-2.91980778121556,
4.74213608943437));
#15938=CARTESIAN_POINT('Ctrl Pts',(-6.72958410590507,-3.16055362161142,
4.80163845366161));
#15939=CARTESIAN_POINT('Ctrl Pts',(-6.922583408066,-3.41255717151317,4.8453962925926));
#15940=CARTESIAN_POINT('Ctrl Pts',(-7.04520229026909,-3.65506744231538,
4.88286085267916));
#15941=CARTESIAN_POINT('Ctrl Pts',(-7.10903827020174,-3.9926759490213,4.92960885619655));
#15942=CARTESIAN_POINT('Ctrl Pts',(-7.032354492376,-4.39667067923105,4.98556279568034));
#15943=CARTESIAN_POINT('Ctrl Pts',(-6.81415974257675,-4.74396102273289,
5.04136211338037));
#15944=CARTESIAN_POINT('Ctrl Pts',(-6.48510242262688,-4.98648342248571,
5.09699623581333));
#15945=CARTESIAN_POINT('Ctrl Pts',(-6.09122164110091,-5.09213718968761,
5.15245506498449));
#15946=CARTESIAN_POINT('Ctrl Pts',(-5.6879156360413,-5.04618557814476,5.20772889788153));
#15947=CARTESIAN_POINT('Ctrl Pts',(-5.20960410281967,-4.79482820495352,
5.28116853491036));
#15948=CARTESIAN_POINT('Ctrl Pts',(-4.85635661256684,-4.18339627204868,
5.37246079310469));
#15949=CARTESIAN_POINT('Ctrl Pts',(-5.04534497366866,-3.36152922837358,
5.4811368047244));
#15950=CARTESIAN_POINT('Ctrl Pts',(-5.62045222073828,-2.97210695679973,
5.57092649482181));
#15951=CARTESIAN_POINT('Ctrl Pts',(-6.14491401311764,-2.95446524901901,
5.64227218329944));
#15952=CARTESIAN_POINT('Ctrl Pts',(-6.55538629310792,-3.09741218079302,
5.70145206897501));
#15953=CARTESIAN_POINT('Ctrl Pts',(-6.90061904209687,-3.43455608810828,
5.76619150175189));
#15954=CARTESIAN_POINT('Ctrl Pts',(-7.05403180026006,-3.93434682913999,
5.83636208061574));
#15955=CARTESIAN_POINT('Ctrl Pts',(-6.95084370870626,-4.44331194962687,
5.90607316768221));
#15956=CARTESIAN_POINT('Ctrl Pts',(-6.61884201115902,-4.83828819326241,
5.97532164622816));
#15957=CARTESIAN_POINT('Ctrl Pts',(-6.14163977231472,-5.02507153362565,
6.04410658214742));
#15958=CARTESIAN_POINT('Ctrl Pts',(-5.67874308979945,-4.96670943531882,
6.10673565115305));
#15959=CARTESIAN_POINT('Ctrl Pts',(-5.32673727495899,-4.74487796933182,
6.16333654805419));
#15960=CARTESIAN_POINT('Ctrl Pts',(-5.10557737295403,-4.44521639081723,
6.21402149420468));
#15961=CARTESIAN_POINT('Ctrl Pts',(-5.00986236436416,-4.08706033297606,
6.26445344628883));
#15962=CARTESIAN_POINT('Ctrl Pts',(-5.05132140869747,-3.72058500062059,
6.31463598386295));
#15963=CARTESIAN_POINT('Ctrl Pts',(-5.22295427342147,-3.39619318419661,
6.36457331207659));
#15964=CARTESIAN_POINT('Ctrl Pts',(-5.49996349858563,-3.15797332202467,
6.41427030413784));
#15965=CARTESIAN_POINT('Ctrl Pts',(-5.843023257891,-3.03825996963253,6.46373244033231));
#15966=CARTESIAN_POINT('Ctrl Pts',(-6.2651798733637,-3.05368284090179,6.52117143934356));
#15967=CARTESIAN_POINT('Ctrl Pts',(-6.69395218073661,-3.29085487418832,
6.58644589644131));
#15968=CARTESIAN_POINT('Ctrl Pts',(-6.9588514090406,-3.77142724594311,6.65940509135759));
#15969=CARTESIAN_POINT('Ctrl Pts',(-6.93289301903251,-4.22410112506723,
6.71983222544231));
#15970=CARTESIAN_POINT('Ctrl Pts',(-6.77106481048377,-4.53615877260298,
6.76796591761938));
#15971=CARTESIAN_POINT('Ctrl Pts',(-6.57088599598262,-4.74749645053629,
6.8079662999785));
#15972=CARTESIAN_POINT('Ctrl Pts',(-6.18196007039062,-4.95496402481898,
6.86778079666891));
#15973=CARTESIAN_POINT('Ctrl Pts',(-5.63200940413013,-4.91297894303413,
6.93919834468442));
#15974=CARTESIAN_POINT('Ctrl Pts',(-5.18963313111942,-4.51545599119052,
7.01814869825501));
#15975=CARTESIAN_POINT('Ctrl Pts',(-5.04266994609727,-4.00519996765647,
7.08893288548598));
#15976=CARTESIAN_POINT('Ctrl Pts',(-5.18994160065279,-3.49569082009585,
7.15948665627275));
#15977=CARTESIAN_POINT('Ctrl Pts',(-5.58406477811046,-3.14370617953113,
7.22985222522876));
#15978=CARTESIAN_POINT('Ctrl Pts',(-6.10419876841606,-3.05543002721108,
7.30007283323036));
#15979=CARTESIAN_POINT('Ctrl Pts',(-6.59085610258569,-3.25712241290123,
7.37019262147636));
#15980=CARTESIAN_POINT('Ctrl Pts',(-6.8952969281062,-3.68642062054244,7.44025632508636));
#15981=CARTESIAN_POINT('Ctrl Pts',(-6.92507910037993,-4.2118623997588,7.51030900497373));
#15982=CARTESIAN_POINT('Ctrl Pts',(-6.67029196164112,-4.6727438878236,7.58039577683535));
#15983=CARTESIAN_POINT('Ctrl Pts',(-6.20902606294958,-4.92782413963266,
7.65056157433059));
#15984=CARTESIAN_POINT('Ctrl Pts',(-5.68175068955988,-4.89838259463549,
7.72085085746158));
#15985=CARTESIAN_POINT('Ctrl Pts',(-5.24995696526907,-4.59224234497362,
7.79130734612191));
#15986=CARTESIAN_POINT('Ctrl Pts',(-5.04653976812282,-4.10189023096155,
7.86197377554524));
#15987=CARTESIAN_POINT('Ctrl Pts',(-5.13553771446182,-3.57654536818086,
7.93289164421975));
#15988=CARTESIAN_POINT('Ctrl Pts',(-5.49167958880606,-3.17757206270347,
8.00410097016463));
#15989=CARTESIAN_POINT('Ctrl Pts',(-6.00820878856796,-3.02820291673281,
8.07564000225066));
#15990=CARTESIAN_POINT('Ctrl Pts',(-6.44062187419601,-3.15261370888403,
8.13556092469148));
#15991=CARTESIAN_POINT('Ctrl Pts',(-6.70861130655355,-3.37965195671477,
8.18369776363854));
#15992=CARTESIAN_POINT('Ctrl Pts',(-6.8937105085998,-3.65581236490976,8.22929135600403));
#15993=CARTESIAN_POINT('Ctrl Pts',(-6.97571459288556,-4.05892831151958,
8.28449961702882));
#15994=CARTESIAN_POINT('Ctrl Pts',(-6.83301647708075,-4.52172879570838,
8.34949564023339));
#15995=CARTESIAN_POINT('Ctrl Pts',(-6.51381452164907,-4.83374162454526,
8.40942447333573));
#15996=CARTESIAN_POINT('Ctrl Pts',(-6.13367096105595,-4.96658596055631,
8.46419547642941));
#15997=CARTESIAN_POINT('Ctrl Pts',(-5.77000769054747,-4.95325944490059,
8.51371979160536));
#15998=CARTESIAN_POINT('Ctrl Pts',(-5.43473421944715,-4.80705755452014,
8.56348049202891));
#15999=CARTESIAN_POINT('Ctrl Pts',(-5.17476962038704,-4.5473411130966,8.6134828902317));
#16000=CARTESIAN_POINT('Ctrl Pts',(-5.02691233865341,-4.20890181210803,
8.66373168353468));
#16001=CARTESIAN_POINT('Ctrl Pts',(-5.01287597198371,-3.83802632501149,
8.71423091550292));
#16002=CARTESIAN_POINT('Ctrl Pts',(-5.13588065841094,-3.48587318149708,
8.76498396862734));
#16003=CARTESIAN_POINT('Ctrl Pts',(-5.38027484984219,-3.20156985271231,
8.81599355960519));
#16004=CARTESIAN_POINT('Ctrl Pts',(-5.71337748308179,-3.0254571982762,8.86726173709343));
#16005=CARTESIAN_POINT('Ctrl Pts',(-6.08966550245643,-2.98274869856715,
8.91878984711541));
#16006=CARTESIAN_POINT('Ctrl Pts',(-6.45733798876018,-3.0812109148485,8.97057858675351));
#16007=CARTESIAN_POINT('Ctrl Pts',(-6.76529910592523,-3.30812336168265,
9.02262792849601));
#16008=CARTESIAN_POINT('Ctrl Pts',(-6.96998046112789,-3.63355675694242,
9.07493719450744));
#16009=CARTESIAN_POINT('Ctrl Pts',(-7.04194989283072,-4.01319995364602,
9.12750500078302));
#16010=CARTESIAN_POINT('Ctrl Pts',(-6.96991048459342,-4.39460760383808,
9.18032929219698));
#16011=CARTESIAN_POINT('Ctrl Pts',(-6.73960211403654,-4.76194359718324,
9.23930488555841));
#16012=CARTESIAN_POINT('Ctrl Pts',(-6.33176853957225,-5.02597941464994,
9.30453505646424));
#16013=CARTESIAN_POINT('Ctrl Pts',(-5.79980377218573,-5.06633098935627,
9.37613051632468));
#16014=CARTESIAN_POINT('Ctrl Pts',(-5.29005475531646,-4.836901018808,9.45115010972279));
#16015=CARTESIAN_POINT('Ctrl Pts',(-4.94827191401131,-4.35650564743655,
9.52964181326016));
#16016=CARTESIAN_POINT('Ctrl Pts',(-4.91327405487842,-3.74129847888372,
9.61164803952703));
#16017=CARTESIAN_POINT('Ctrl Pts',(-5.21254904956895,-3.19880095424663,
9.69412425066449));
#16018=CARTESIAN_POINT('Ctrl Pts',(-5.75755518053287,-2.89705290752891,
9.77704206923956));
#16019=CARTESIAN_POINT('Ctrl Pts',(-6.38261532053777,-2.93174547355756,
9.86037047436186));
#16020=CARTESIAN_POINT('Ctrl Pts',(-6.89571246871018,-3.29533246954376,
9.9440760489684));
#16021=CARTESIAN_POINT('Ctrl Pts',(-7.13766462222267,-3.87856431327716,
10.0281231253342));
#16022=CARTESIAN_POINT('Ctrl Pts',(-7.03181307520858,-4.50336859593469,
10.112474009291));
#16023=CARTESIAN_POINT('Ctrl Pts',(-6.60841405754483,-4.9775421382096,10.1970892234063));
#16024=CARTESIAN_POINT('Ctrl Pts',(-5.99601356400164,-5.15419586953956,
10.2819277209876));
#16025=CARTESIAN_POINT('Ctrl Pts',(-5.38220054085499,-4.97753568370925,
10.3669471364924));
#16026=CARTESIAN_POINT('Ctrl Pts',(-4.95580917322647,-4.50058383383181,
10.4521040148979));
#16027=CARTESIAN_POINT('Ctrl Pts',(-4.84845524689304,-3.86918295104257,
10.5373541217208));
#16028=CARTESIAN_POINT('Ctrl Pts',(-5.09367725879538,-3.27712852401529,
10.6226526455382));
#16029=CARTESIAN_POINT('Ctrl Pts',(-5.6163401918585,-2.90630478068196,10.7079544990261));
#16030=CARTESIAN_POINT('Ctrl Pts',(-6.25592072702474,-2.87046899980689,
10.7932145516894));
#16031=CARTESIAN_POINT('Ctrl Pts',(-6.81586294759382,-3.18009679237689,
10.8783879977619));
#16032=CARTESIAN_POINT('Ctrl Pts',(-7.124955642463,-3.73939634942269,10.963430385322));
#16033=CARTESIAN_POINT('Ctrl Pts',(-7.08867264951758,-4.37593520057008,
11.0482983435205));
#16034=CARTESIAN_POINT('Ctrl Pts',(-6.72062823969146,-4.89450906450982,
11.1329488746335));
#16035=CARTESIAN_POINT('Ctrl Pts',(-6.13472454520284,-5.136799701332,11.217341733611));
#16036=CARTESIAN_POINT('Ctrl Pts',(-5.51200536776972,-5.03087324497862,
11.3014349939178));
#16037=CARTESIAN_POINT('Ctrl Pts',(-5.04306930328679,-4.6109089567958,11.3851957518917));
#16038=CARTESIAN_POINT('Ctrl Pts',(-4.92780437314592,-4.2103503377694,11.4407823887583));
#16039=CARTESIAN_POINT('Ctrl Pts',(-4.92777733020741,-4.00946826990451,
11.4685145081939));
#16040=CARTESIAN_POINT('Origin',(-5.,-4.,11.4));
#16041=CARTESIAN_POINT('Origin',(-5.,-4.,11.4));
#16042=CARTESIAN_POINT('Origin',(-5.,-4.,2.7));
#22304=UNCERTAINTY_MEASURE_WITH_UNIT(LENGTH_MEASURE(0.001),#22395,
'DISTANCE_ACCURACY_VALUE',
'Maximum model space distance between geometric entities at asserted c
onnectivities');
#22343=UNCERTAINTY_MEASURE_WITH_UNIT(LENGTH_MEASURE(0.001),#22395,
'DISTANCE_ACCURACY_VALUE',
'Maximum model space distance between geometric entities at asserted c
onnectivities');
#22355=(
GEOMETRIC_REPRESENTATION_CONTEXT(3)
GLOBAL_UNCERTAINTY_ASSIGNED_CONTEXT((#22304))
GLOBAL_UNIT_ASSIGNED_CONTEXT((#22395,#22397,#22398))
REPRESENTATION_CONTEXT('','3D')
);
#22394=(
GEOMETRIC_REPRESENTATION_CONTEXT(3)
GLOBAL_UNCERTAINTY_ASSIGNED_CONTEXT((#22343))
GLOBAL_UNIT_ASSIGNED_CONTEXT((#22395,#22397,#22398))
REPRESENTATION_CONTEXT('','3D')
);
#22395=(
LENGTH_UNIT()
NAMED_UNIT(*)
SI_UNIT(.CENTI.,.METRE.)
);
#22397=(
NAMED_UNIT(*)
PLANE_ANGLE_UNIT()
SI_UNIT($,.RADIAN.)
);
#22398=(
NAMED_UNIT(*)
SI_UNIT($,.STERADIAN.)
SOLID_ANGLE_UNIT()
);
#22410=SHAPE_DEFINITION_REPRESENTATION(#22460,#22649);
#22460=PRODUCT_DEFINITION_SHAPE('',$,#22700);
#22649=SHAPE_REPRESENTATION('',(#10013),#22355);
#22688=PRODUCT_DEFINITION_CONTEXT('part definition',#22840,'design');
#22700=PRODUCT_DEFINITION('Installed compression spring',
'Installed compression spring',#22750,#22688);
#22750=PRODUCT_DEFINITION_FORMATION('',$,#22853);
#22840=APPLICATION_CONTEXT(
'Core Data for Automotive Mechanical Design Process');
#22841=PRODUCT_CONTEXT('part definition',#22840,'mechanical');
#22853=PRODUCT('Installed compression spring',
'Installed compression spring','Installed compression spring',(#22841));
#22955=COLOUR_RGB('Grey',0.48,0.52,0.57);
#22956=FILL_AREA_STYLE_COLOUR('',#22955);
#22957=FILL_AREA_STYLE('',(#22956));
#22958=SURFACE_STYLE_FILL_AREA(#22957);
#22959=SURFACE_SIDE_STYLE('',(#22958));
#22960=SURFACE_STYLE_USAGE(.BOTH.,#22959);
#22961=PRESENTATION_STYLE_ASSIGNMENT((#22960));
ENDSEC;
END-ISO-10303-21;
